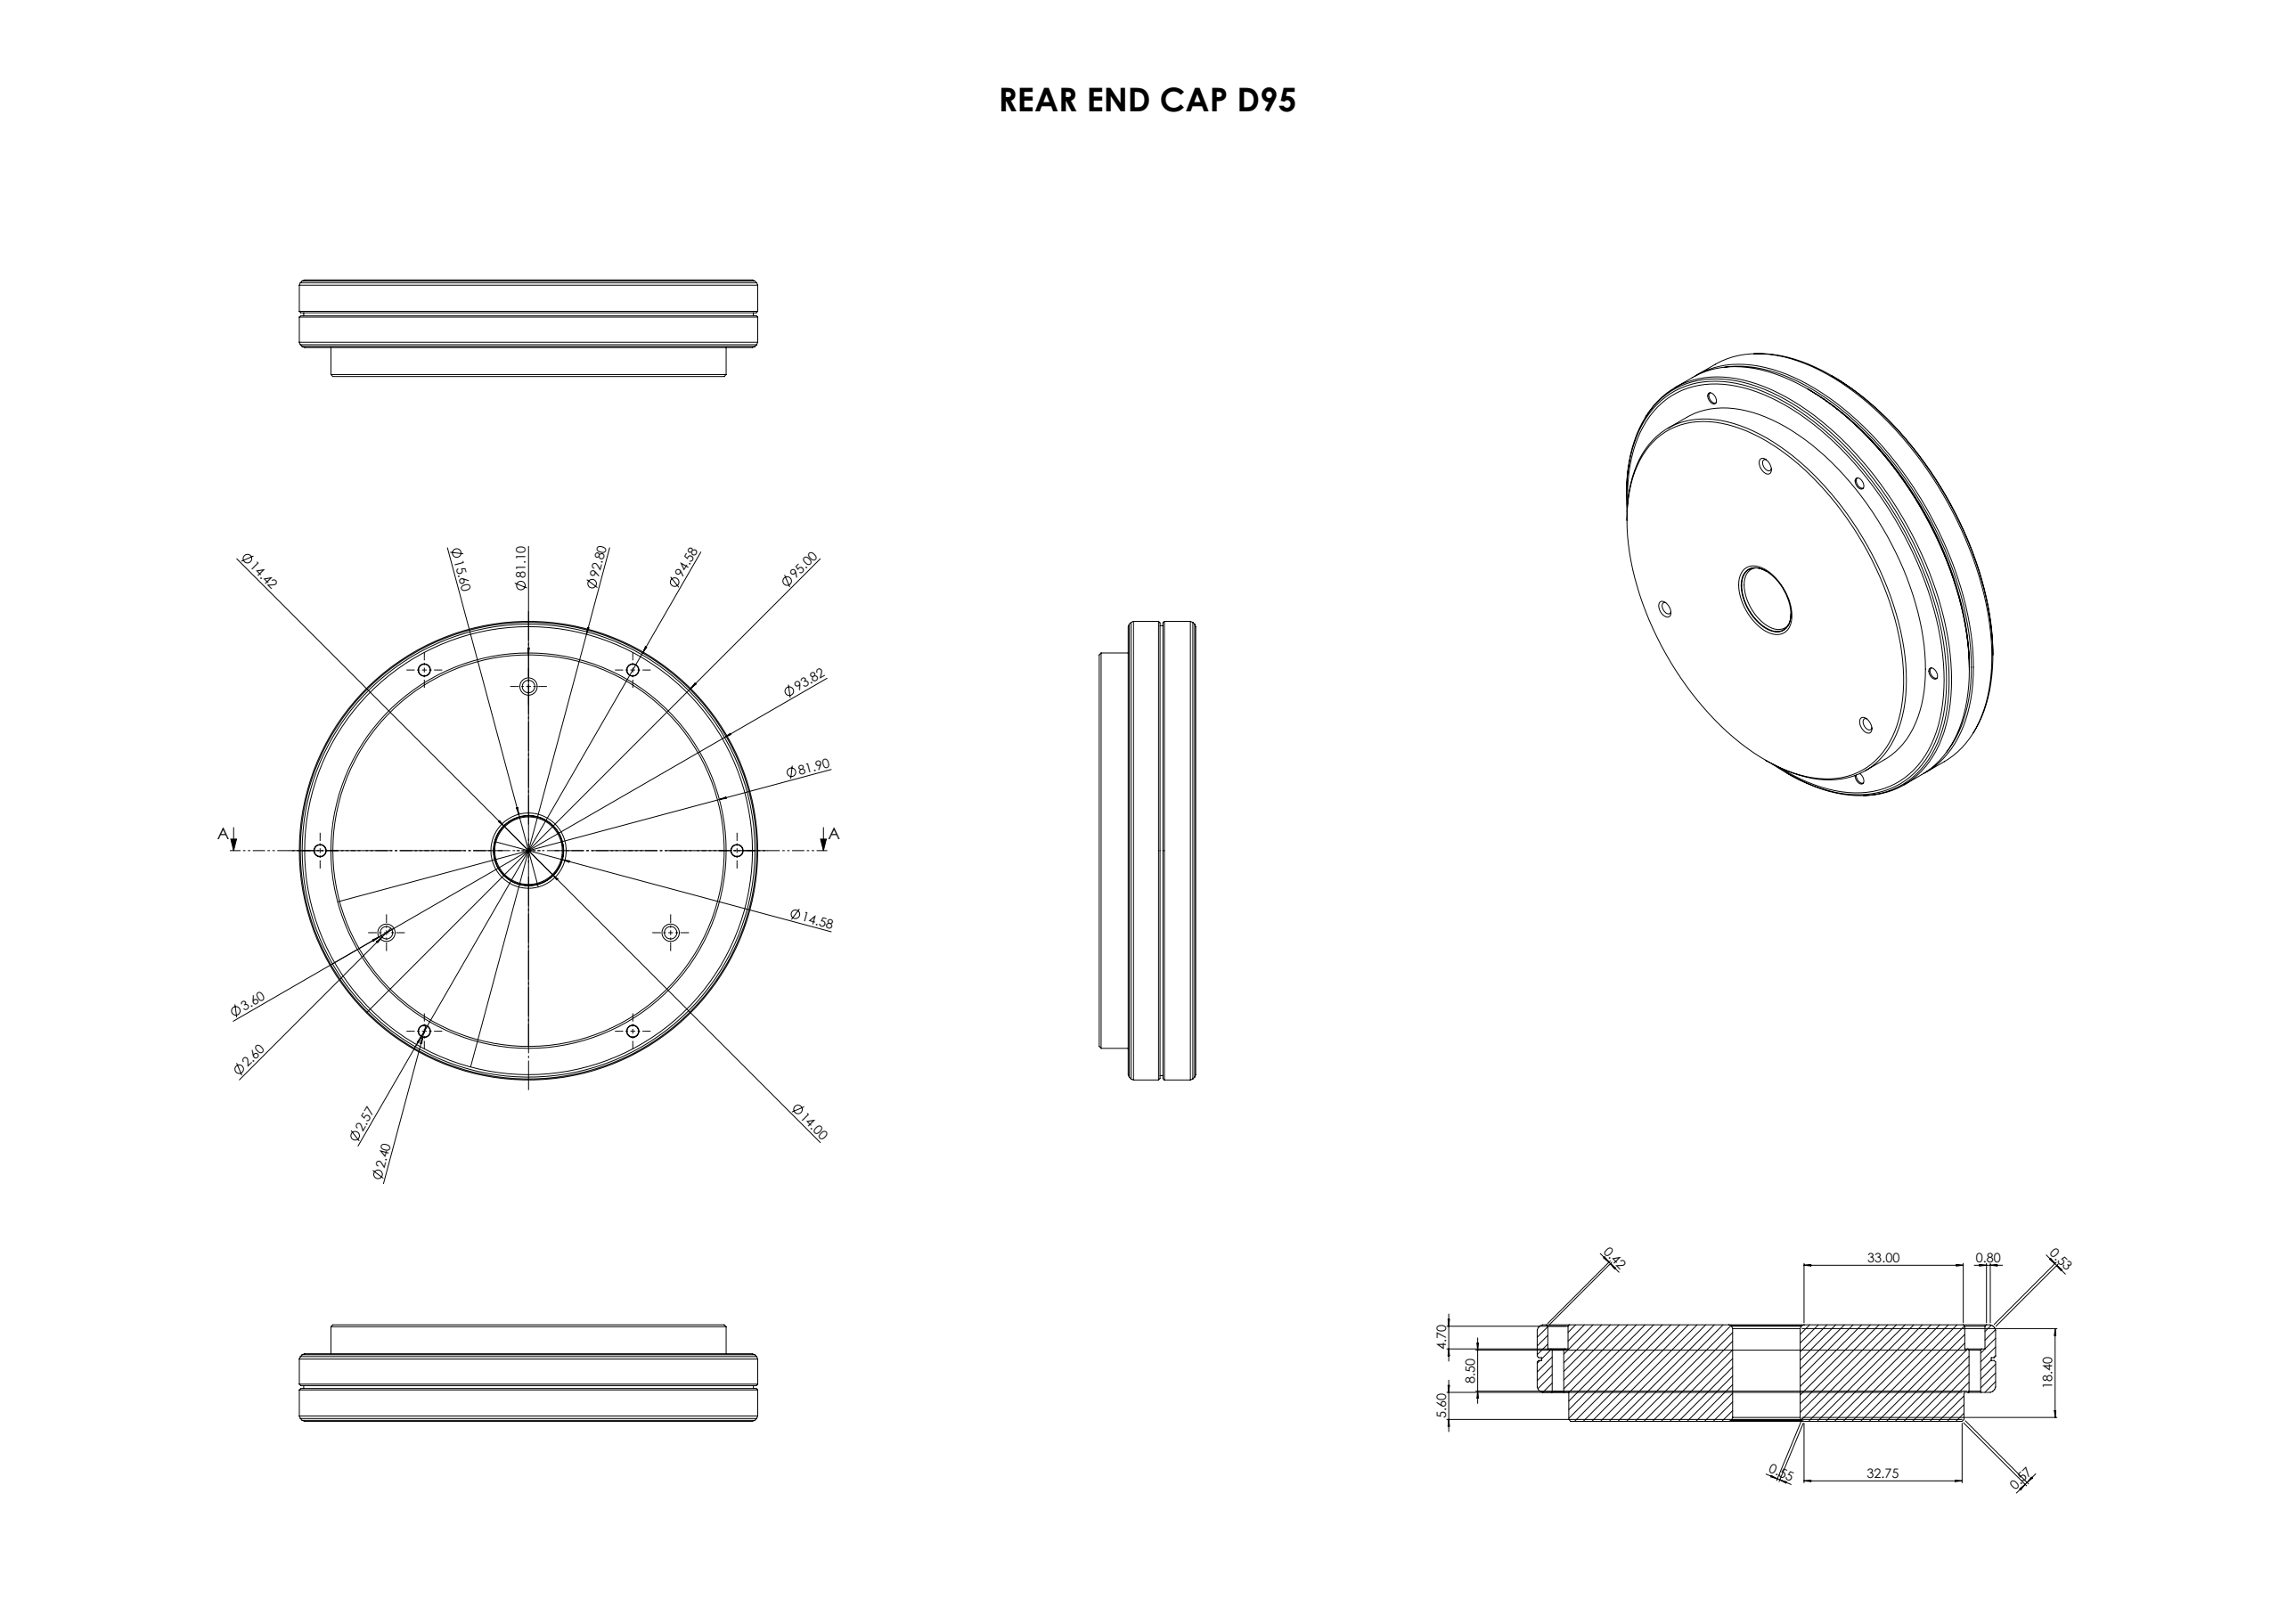
ISO-10303-21;
HEADER;
/* Generated by software containing ST-Developer
 * from STEP Tools, Inc. (www.steptools.com) 
 */

FILE_DESCRIPTION(
/* description */ (''),
/* implementation_level */ '2;1');

FILE_NAME(
/* name */ '01_Rear_End_Cap_D95.step',
/* time_stamp */ '2026-10-19T23:00:43-07:00',
/* author */ (''),
/* organization */ (''),
/* preprocessor_version */ 'ST-DEVELOPER v20.2',
/* originating_system */ 'Autodesk Translation Framework v15.15.0.0',
/* authorisation */ '');

FILE_SCHEMA (('AUTOMOTIVE_DESIGN { 1 0 10303 214 3 1 1 }'));
ENDSEC;

DATA;
#10=MECHANICAL_DESIGN_GEOMETRIC_PRESENTATION_REPRESENTATION('',(#996),#55002);
#956=SHAPE_REPRESENTATION_RELATIONSHIP('SRR','None',#55104,#976);
#976=ADVANCED_BREP_SHAPE_REPRESENTATION('',(#1016),#54982);
#996=STYLED_ITEM('',(#55372),#1016);
#1016=MANIFOLD_SOLID_BREP('Rear End Cap',#24529);
#1036=FACE_BOUND('',#3782,.T.);
#1037=FACE_BOUND('',#3783,.T.);
#1038=FACE_BOUND('',#3784,.T.);
#1039=FACE_BOUND('',#3785,.T.);
#1040=FACE_BOUND('',#3786,.T.);
#1041=FACE_BOUND('',#3787,.T.);
#1042=FACE_BOUND('',#3788,.T.);
#1043=FACE_BOUND('',#3791,.T.);
#1044=FACE_BOUND('',#3792,.T.);
#1045=FACE_BOUND('',#3793,.T.);
#1046=FACE_BOUND('',#3794,.T.);
#1047=FACE_BOUND('',#3795,.T.);
#1048=FACE_BOUND('',#3796,.T.);
#1049=FACE_BOUND('',#3797,.T.);
#1050=FACE_BOUND('',#3806,.T.);
#1051=FACE_BOUND('',#3807,.T.);
#1052=FACE_BOUND('',#3808,.T.);
#1053=FACE_BOUND('',#3809,.T.);
#1054=FACE_BOUND('',#3826,.T.);
#1055=FACE_BOUND('',#3829,.T.);
#1056=FACE_BOUND('',#3844,.T.);
#1057=FACE_BOUND('',#3849,.T.);
#1058=FACE_BOUND('',#3854,.T.);
#1059=FACE_BOUND('',#3859,.T.);
#1060=FACE_BOUND('',#3864,.T.);
#1061=FACE_BOUND('',#3869,.T.);
#1276=PLANE('',#24785);
#1277=PLANE('',#24795);
#1278=PLANE('',#24819);
#1279=PLANE('',#24861);
#1280=PLANE('',#24865);
#1281=PLANE('',#24889);
#1282=PLANE('',#24896);
#1283=PLANE('',#24903);
#1284=PLANE('',#24910);
#1285=PLANE('',#24917);
#1286=PLANE('',#24924);
#1952=CYLINDRICAL_SURFACE('',#24778,4.75);
#1953=CYLINDRICAL_SURFACE('',#24810,0.7);
#1954=CYLINDRICAL_SURFACE('',#24827,0.21);
#1955=CYLINDRICAL_SURFACE('',#24832,0.21);
#1956=CYLINDRICAL_SURFACE('',#24837,0.21);
#1957=CYLINDRICAL_SURFACE('',#24842,0.21);
#1958=CYLINDRICAL_SURFACE('',#24847,0.21);
#1959=CYLINDRICAL_SURFACE('',#24852,0.21);
#1960=CYLINDRICAL_SURFACE('',#24857,4.75);
#1961=CYLINDRICAL_SURFACE('',#24867,4.66);
#1962=CYLINDRICAL_SURFACE('',#24870,0.13);
#1963=CYLINDRICAL_SURFACE('',#24875,0.13);
#1964=CYLINDRICAL_SURFACE('',#24880,0.13);
#1965=CYLINDRICAL_SURFACE('',#24885,0.12);
#1966=CYLINDRICAL_SURFACE('',#24892,0.12);
#1967=CYLINDRICAL_SURFACE('',#24899,0.12);
#1968=CYLINDRICAL_SURFACE('',#24906,0.12);
#1969=CYLINDRICAL_SURFACE('',#24913,0.12);
#1970=CYLINDRICAL_SURFACE('',#24920,0.12);
#1971=CYLINDRICAL_SURFACE('',#24928,4.095);
#2412=FACE_OUTER_BOUND('',#3776,.T.);
#2413=FACE_OUTER_BOUND('',#3777,.T.);
#2414=FACE_OUTER_BOUND('',#3778,.T.);
#2415=FACE_OUTER_BOUND('',#3779,.T.);
#2416=FACE_OUTER_BOUND('',#3780,.T.);
#2417=FACE_OUTER_BOUND('',#3781,.T.);
#2418=FACE_OUTER_BOUND('',#3789,.T.);
#2419=FACE_OUTER_BOUND('',#3790,.T.);
#2420=FACE_OUTER_BOUND('',#3798,.T.);
#2421=FACE_OUTER_BOUND('',#3799,.T.);
#2422=FACE_OUTER_BOUND('',#3800,.T.);
#2423=FACE_OUTER_BOUND('',#3801,.T.);
#2424=FACE_OUTER_BOUND('',#3802,.T.);
#2425=FACE_OUTER_BOUND('',#3803,.T.);
#2426=FACE_OUTER_BOUND('',#3804,.T.);
#2427=FACE_OUTER_BOUND('',#3805,.T.);
#2428=FACE_OUTER_BOUND('',#3810,.T.);
#2429=FACE_OUTER_BOUND('',#3811,.T.);
#2430=FACE_OUTER_BOUND('',#3812,.T.);
#2431=FACE_OUTER_BOUND('',#3813,.T.);
#2432=FACE_OUTER_BOUND('',#3814,.T.);
#2433=FACE_OUTER_BOUND('',#3815,.T.);
#2434=FACE_OUTER_BOUND('',#3816,.T.);
#2435=FACE_OUTER_BOUND('',#3817,.T.);
#2436=FACE_OUTER_BOUND('',#3818,.T.);
#2437=FACE_OUTER_BOUND('',#3819,.T.);
#2438=FACE_OUTER_BOUND('',#3820,.T.);
#2439=FACE_OUTER_BOUND('',#3821,.T.);
#2440=FACE_OUTER_BOUND('',#3822,.T.);
#2441=FACE_OUTER_BOUND('',#3823,.T.);
#2442=FACE_OUTER_BOUND('',#3824,.T.);
#2443=FACE_OUTER_BOUND('',#3825,.T.);
#2444=FACE_OUTER_BOUND('',#3827,.T.);
#2445=FACE_OUTER_BOUND('',#3828,.T.);
#2446=FACE_OUTER_BOUND('',#3830,.T.);
#2447=FACE_OUTER_BOUND('',#3831,.T.);
#2448=FACE_OUTER_BOUND('',#3832,.T.);
#2449=FACE_OUTER_BOUND('',#3833,.T.);
#2450=FACE_OUTER_BOUND('',#3834,.T.);
#2451=FACE_OUTER_BOUND('',#3835,.T.);
#2452=FACE_OUTER_BOUND('',#3836,.T.);
#2453=FACE_OUTER_BOUND('',#3837,.T.);
#2454=FACE_OUTER_BOUND('',#3838,.T.);
#2455=FACE_OUTER_BOUND('',#3839,.T.);
#2456=FACE_OUTER_BOUND('',#3840,.T.);
#2457=FACE_OUTER_BOUND('',#3841,.T.);
#2458=FACE_OUTER_BOUND('',#3842,.T.);
#2459=FACE_OUTER_BOUND('',#3843,.T.);
#2460=FACE_OUTER_BOUND('',#3845,.T.);
#2461=FACE_OUTER_BOUND('',#3846,.T.);
#2462=FACE_OUTER_BOUND('',#3847,.T.);
#2463=FACE_OUTER_BOUND('',#3848,.T.);
#2464=FACE_OUTER_BOUND('',#3850,.T.);
#2465=FACE_OUTER_BOUND('',#3851,.T.);
#2466=FACE_OUTER_BOUND('',#3852,.T.);
#2467=FACE_OUTER_BOUND('',#3853,.T.);
#2468=FACE_OUTER_BOUND('',#3855,.T.);
#2469=FACE_OUTER_BOUND('',#3856,.T.);
#2470=FACE_OUTER_BOUND('',#3857,.T.);
#2471=FACE_OUTER_BOUND('',#3858,.T.);
#2472=FACE_OUTER_BOUND('',#3860,.T.);
#2473=FACE_OUTER_BOUND('',#3861,.T.);
#2474=FACE_OUTER_BOUND('',#3862,.T.);
#2475=FACE_OUTER_BOUND('',#3863,.T.);
#2476=FACE_OUTER_BOUND('',#3865,.T.);
#2477=FACE_OUTER_BOUND('',#3866,.T.);
#2478=FACE_OUTER_BOUND('',#3867,.T.);
#2479=FACE_OUTER_BOUND('',#3868,.T.);
#2480=FACE_OUTER_BOUND('',#3870,.T.);
#2481=FACE_OUTER_BOUND('',#3871,.T.);
#3776=EDGE_LOOP('',(#15886,#15887,#15888,#15889,#15890));
#3777=EDGE_LOOP('',(#15891,#15892,#15893,#15894));
#3778=EDGE_LOOP('',(#15895,#15896,#15897,#15898,#15899));
#3779=EDGE_LOOP('',(#15900,#15901,#15902,#15903));
#3780=EDGE_LOOP('',(#15904,#15905,#15906,#15907));
#3781=EDGE_LOOP('',(#15908));
#3782=EDGE_LOOP('',(#15909));
#3783=EDGE_LOOP('',(#15910));
#3784=EDGE_LOOP('',(#15911));
#3785=EDGE_LOOP('',(#15912));
#3786=EDGE_LOOP('',(#15913));
#3787=EDGE_LOOP('',(#15914));
#3788=EDGE_LOOP('',(#15915));
#3789=EDGE_LOOP('',(#15916,#15917,#15918,#15919));
#3790=EDGE_LOOP('',(#15920));
#3791=EDGE_LOOP('',(#15921));
#3792=EDGE_LOOP('',(#15922));
#3793=EDGE_LOOP('',(#15923));
#3794=EDGE_LOOP('',(#15924));
#3795=EDGE_LOOP('',(#15925));
#3796=EDGE_LOOP('',(#15926));
#3797=EDGE_LOOP('',(#15927));
#3798=EDGE_LOOP('',(#15928,#15929,#15930,#15931));
#3799=EDGE_LOOP('',(#15932,#15933,#15934,#15935));
#3800=EDGE_LOOP('',(#15936,#15937,#15938,#15939,#15940));
#3801=EDGE_LOOP('',(#15941,#15942,#15943,#15944,#15945,#15946));
#3802=EDGE_LOOP('',(#15947,#15948,#15949,#15950,#15951));
#3803=EDGE_LOOP('',(#15952,#15953,#15954,#15955));
#3804=EDGE_LOOP('',(#15956,#15957,#15958,#15959));
#3805=EDGE_LOOP('',(#15960));
#3806=EDGE_LOOP('',(#15961));
#3807=EDGE_LOOP('',(#15962));
#3808=EDGE_LOOP('',(#15963));
#3809=EDGE_LOOP('',(#15964));
#3810=EDGE_LOOP('',(#15965,#15966,#15967,#15968,#15969));
#3811=EDGE_LOOP('',(#15970,#15971,#15972,#15973,#15974));
#3812=EDGE_LOOP('',(#15975,#15976,#15977,#15978,#15979));
#3813=EDGE_LOOP('',(#15980,#15981,#15982,#15983,#15984));
#3814=EDGE_LOOP('',(#15985,#15986,#15987,#15988,#15989));
#3815=EDGE_LOOP('',(#15990,#15991,#15992,#15993,#15994));
#3816=EDGE_LOOP('',(#15995,#15996,#15997,#15998,#15999));
#3817=EDGE_LOOP('',(#16000,#16001,#16002,#16003,#16004));
#3818=EDGE_LOOP('',(#16005,#16006,#16007,#16008,#16009));
#3819=EDGE_LOOP('',(#16010,#16011,#16012,#16013,#16014));
#3820=EDGE_LOOP('',(#16015,#16016,#16017,#16018,#16019));
#3821=EDGE_LOOP('',(#16020,#16021,#16022,#16023,#16024));
#3822=EDGE_LOOP('',(#16025,#16026,#16027,#16028,#16029));
#3823=EDGE_LOOP('',(#16030,#16031,#16032,#16033,#16034));
#3824=EDGE_LOOP('',(#16035,#16036,#16037,#16038));
#3825=EDGE_LOOP('',(#16039));
#3826=EDGE_LOOP('',(#16040));
#3827=EDGE_LOOP('',(#16041,#16042,#16043,#16044));
#3828=EDGE_LOOP('',(#16045));
#3829=EDGE_LOOP('',(#16046));
#3830=EDGE_LOOP('',(#16047,#16048,#16049,#16050));
#3831=EDGE_LOOP('',(#16051,#16052,#16053));
#3832=EDGE_LOOP('',(#16054,#16055,#16056,#16057));
#3833=EDGE_LOOP('',(#16058,#16059,#16060,#16061));
#3834=EDGE_LOOP('',(#16062,#16063,#16064));
#3835=EDGE_LOOP('',(#16065,#16066,#16067,#16068));
#3836=EDGE_LOOP('',(#16069,#16070,#16071,#16072));
#3837=EDGE_LOOP('',(#16073,#16074,#16075));
#3838=EDGE_LOOP('',(#16076,#16077,#16078,#16079));
#3839=EDGE_LOOP('',(#16080,#16081,#16082,#16083));
#3840=EDGE_LOOP('',(#16084,#16085,#16086,#16087));
#3841=EDGE_LOOP('',(#16088,#16089,#16090,#16091));
#3842=EDGE_LOOP('',(#16092,#16093,#16094,#16095));
#3843=EDGE_LOOP('',(#16096));
#3844=EDGE_LOOP('',(#16097));
#3845=EDGE_LOOP('',(#16098,#16099,#16100,#16101));
#3846=EDGE_LOOP('',(#16102,#16103,#16104,#16105));
#3847=EDGE_LOOP('',(#16106,#16107,#16108,#16109));
#3848=EDGE_LOOP('',(#16110));
#3849=EDGE_LOOP('',(#16111));
#3850=EDGE_LOOP('',(#16112,#16113,#16114,#16115));
#3851=EDGE_LOOP('',(#16116,#16117,#16118,#16119));
#3852=EDGE_LOOP('',(#16120,#16121,#16122,#16123));
#3853=EDGE_LOOP('',(#16124));
#3854=EDGE_LOOP('',(#16125));
#3855=EDGE_LOOP('',(#16126,#16127,#16128,#16129));
#3856=EDGE_LOOP('',(#16130,#16131,#16132,#16133));
#3857=EDGE_LOOP('',(#16134,#16135,#16136,#16137));
#3858=EDGE_LOOP('',(#16138));
#3859=EDGE_LOOP('',(#16139));
#3860=EDGE_LOOP('',(#16140,#16141,#16142,#16143));
#3861=EDGE_LOOP('',(#16144,#16145,#16146,#16147));
#3862=EDGE_LOOP('',(#16148,#16149,#16150,#16151));
#3863=EDGE_LOOP('',(#16152));
#3864=EDGE_LOOP('',(#16153));
#3865=EDGE_LOOP('',(#16154,#16155,#16156,#16157));
#3866=EDGE_LOOP('',(#16158,#16159,#16160,#16161));
#3867=EDGE_LOOP('',(#16162,#16163,#16164,#16165));
#3868=EDGE_LOOP('',(#16166));
#3869=EDGE_LOOP('',(#16167));
#3870=EDGE_LOOP('',(#16168,#16169,#16170,#16171,#16172));
#3871=EDGE_LOOP('',(#16173,#16174,#16175,#16176,#16177));
#5380=LINE('',#33875,#7201);
#5381=LINE('',#33881,#7202);
#5382=LINE('',#33886,#7203);
#5383=LINE('',#33891,#7204);
#5384=LINE('',#33895,#7205);
#5385=LINE('',#33914,#7206);
#5386=LINE('',#33934,#7207);
#5387=LINE('',#33937,#7208);
#5388=LINE('',#33941,#7209);
#5389=LINE('',#33950,#7210);
#5390=LINE('',#33954,#7211);
#5391=LINE('',#33957,#7212);
#5392=LINE('',#33961,#7213);
#5393=LINE('',#33974,#7214);
#5394=LINE('',#33981,#7215);
#5395=LINE('',#33984,#7216);
#5396=LINE('',#33991,#7217);
#5397=LINE('',#33994,#7218);
#5398=LINE('',#34001,#7219);
#5399=LINE('',#34004,#7220);
#5400=LINE('',#34011,#7221);
#5401=LINE('',#34014,#7222);
#5402=LINE('',#34021,#7223);
#5403=LINE('',#34024,#7224);
#5404=LINE('',#34031,#7225);
#5405=LINE('',#34034,#7226);
#5406=LINE('',#34040,#7227);
#5407=LINE('',#34044,#7228);
#5408=LINE('',#34051,#7229);
#5409=LINE('',#34057,#7230);
#5410=LINE('',#34061,#7231);
#5411=LINE('',#34065,#7232);
#5412=LINE('',#34068,#7233);
#5413=LINE('',#34072,#7234);
#5414=LINE('',#34076,#7235);
#5415=LINE('',#34079,#7236);
#5416=LINE('',#34083,#7237);
#5417=LINE('',#34087,#7238);
#5418=LINE('',#34090,#7239);
#5419=LINE('',#34093,#7240);
#5420=LINE('',#34097,#7241);
#5421=LINE('',#34101,#7242);
#5422=LINE('',#34106,#7243);
#5423=LINE('',#34110,#7244);
#5424=LINE('',#34114,#7245);
#5425=LINE('',#34119,#7246);
#5426=LINE('',#34123,#7247);
#5427=LINE('',#34127,#7248);
#5428=LINE('',#34132,#7249);
#5429=LINE('',#34136,#7250);
#5430=LINE('',#34140,#7251);
#5431=LINE('',#34145,#7252);
#5432=LINE('',#34149,#7253);
#5433=LINE('',#34153,#7254);
#5434=LINE('',#34158,#7255);
#5435=LINE('',#34162,#7256);
#5436=LINE('',#34166,#7257);
#5437=LINE('',#34171,#7258);
#5438=LINE('',#34176,#7259);
#7201=VECTOR('',#27204,4.7393933982822);
#7202=VECTOR('',#27211,4.71);
#7203=VECTOR('',#27218,4.75);
#7204=VECTOR('',#27223,4.6656066017178);
#7205=VECTOR('',#27228,4.71);
#7206=VECTOR('',#27249,4.6656066017178);
#7207=VECTOR('',#27272,0.754393398282202);
#7208=VECTOR('',#27275,0.725);
#7209=VECTOR('',#27280,0.710606601717798);
#7210=VECTOR('',#27291,0.7);
#7211=VECTOR('',#27296,0.710606601717798);
#7212=VECTOR('',#27299,0.725);
#7213=VECTOR('',#27304,0.754393398282202);
#7214=VECTOR('',#27319,0.225);
#7215=VECTOR('',#27328,0.21);
#7216=VECTOR('',#27331,0.225);
#7217=VECTOR('',#27340,0.21);
#7218=VECTOR('',#27343,0.225);
#7219=VECTOR('',#27352,0.21);
#7220=VECTOR('',#27355,0.225);
#7221=VECTOR('',#27364,0.21);
#7222=VECTOR('',#27367,0.225);
#7223=VECTOR('',#27376,0.21);
#7224=VECTOR('',#27379,0.225);
#7225=VECTOR('',#27388,0.21);
#7226=VECTOR('',#27391,4.7393933982822);
#7227=VECTOR('',#27398,4.75);
#7228=VECTOR('',#27403,4.735);
#7229=VECTOR('',#27412,4.735);
#7230=VECTOR('',#27421,4.66);
#7231=VECTOR('',#27424,0.0649999999999999);
#7232=VECTOR('',#27429,0.13);
#7233=VECTOR('',#27434,0.18);
#7234=VECTOR('',#27437,0.0649999999999999);
#7235=VECTOR('',#27442,0.13);
#7236=VECTOR('',#27447,0.18);
#7237=VECTOR('',#27450,0.065);
#7238=VECTOR('',#27455,0.13);
#7239=VECTOR('',#27460,0.18);
#7240=VECTOR('',#27463,0.1325);
#7241=VECTOR('',#27468,0.12);
#7242=VECTOR('',#27473,0.1325);
#7243=VECTOR('',#27480,0.1325);
#7244=VECTOR('',#27485,0.12);
#7245=VECTOR('',#27490,0.1325);
#7246=VECTOR('',#27497,0.1325);
#7247=VECTOR('',#27502,0.12);
#7248=VECTOR('',#27507,0.1325);
#7249=VECTOR('',#27514,0.132499999999999);
#7250=VECTOR('',#27519,0.12);
#7251=VECTOR('',#27524,0.132499999999999);
#7252=VECTOR('',#27531,0.1325);
#7253=VECTOR('',#27536,0.12);
#7254=VECTOR('',#27541,0.1325);
#7255=VECTOR('',#27548,0.1325);
#7256=VECTOR('',#27553,0.12);
#7257=VECTOR('',#27558,0.1325);
#7258=VECTOR('',#27565,4.075);
#7259=VECTOR('',#27572,4.095);
#9022=CIRCLE('',#24773,4.7287867965644);
#9023=CIRCLE('',#24774,4.75);
#9024=CIRCLE('',#24775,4.75);
#9025=CIRCLE('',#24777,4.6912132034356);
#9026=CIRCLE('',#24779,4.75);
#9027=CIRCLE('',#24781,4.6912132034356);
#9028=CIRCLE('',#24782,4.64);
#9029=CIRCLE('',#24784,4.7287867965644);
#9030=CIRCLE('',#24786,4.095);
#9031=CIRCLE('',#24787,0.128333333333333);
#9032=CIRCLE('',#24788,0.128333333333333);
#9033=CIRCLE('',#24789,0.128333333333333);
#9034=CIRCLE('',#24790,0.128333333333333);
#9035=CIRCLE('',#24791,0.128333333333334);
#9036=CIRCLE('',#24792,0.128333333333333);
#9037=CIRCLE('',#24794,4.64);
#9038=CIRCLE('',#24796,0.78);
#9039=CIRCLE('',#24797,0.24);
#9040=CIRCLE('',#24798,0.24);
#9041=CIRCLE('',#24799,0.24);
#9042=CIRCLE('',#24800,0.24);
#9043=CIRCLE('',#24801,0.24);
#9044=CIRCLE('',#24802,0.24);
#9045=CIRCLE('',#24804,0.728786796564404);
#9046=CIRCLE('',#24806,0.721213203435596);
#9047=CIRCLE('',#24808,0.7);
#9048=CIRCLE('',#24809,0.7);
#9049=CIRCLE('',#24811,0.7);
#9050=CIRCLE('',#24812,0.7);
#9051=CIRCLE('',#24814,0.721213203435596);
#9052=CIRCLE('',#24816,0.728786796564404);
#9053=CIRCLE('',#24818,0.78);
#9054=CIRCLE('',#24820,4.055);
#9055=CIRCLE('',#24821,0.18);
#9056=CIRCLE('',#24822,0.18);
#9057=CIRCLE('',#24823,0.18);
#9058=CIRCLE('',#24825,0.21);
#9059=CIRCLE('',#24826,0.21);
#9060=CIRCLE('',#24828,0.21);
#9061=CIRCLE('',#24830,0.21);
#9062=CIRCLE('',#24831,0.21);
#9063=CIRCLE('',#24833,0.21);
#9064=CIRCLE('',#24835,0.21);
#9065=CIRCLE('',#24836,0.21);
#9066=CIRCLE('',#24838,0.21);
#9067=CIRCLE('',#24840,0.21);
#9068=CIRCLE('',#24841,0.21);
#9069=CIRCLE('',#24843,0.21);
#9070=CIRCLE('',#24845,0.21);
#9071=CIRCLE('',#24846,0.21);
#9072=CIRCLE('',#24848,0.21);
#9073=CIRCLE('',#24850,0.21);
#9074=CIRCLE('',#24851,0.21);
#9075=CIRCLE('',#24853,0.21);
#9076=CIRCLE('',#24855,4.75);
#9077=CIRCLE('',#24856,4.75);
#9078=CIRCLE('',#24858,4.75);
#9079=CIRCLE('',#24860,4.72);
#9080=CIRCLE('',#24862,4.66);
#9081=CIRCLE('',#24864,4.72);
#9082=CIRCLE('',#24866,4.66);
#9083=CIRCLE('',#24869,0.13);
#9084=CIRCLE('',#24871,0.13);
#9085=CIRCLE('',#24874,0.13);
#9086=CIRCLE('',#24876,0.13);
#9087=CIRCLE('',#24879,0.13);
#9088=CIRCLE('',#24881,0.13);
#9089=CIRCLE('',#24884,0.12);
#9090=CIRCLE('',#24886,0.12);
#9091=CIRCLE('',#24888,0.145);
#9092=CIRCLE('',#24891,0.12);
#9093=CIRCLE('',#24893,0.12);
#9094=CIRCLE('',#24895,0.145);
#9095=CIRCLE('',#24898,0.12);
#9096=CIRCLE('',#24900,0.12);
#9097=CIRCLE('',#24902,0.145);
#9098=CIRCLE('',#24905,0.12);
#9099=CIRCLE('',#24907,0.12);
#9100=CIRCLE('',#24909,0.145);
#9101=CIRCLE('',#24912,0.12);
#9102=CIRCLE('',#24914,0.12);
#9103=CIRCLE('',#24916,0.145);
#9104=CIRCLE('',#24919,0.12);
#9105=CIRCLE('',#24921,0.12);
#9106=CIRCLE('',#24923,0.145);
#9107=CIRCLE('',#24926,4.095);
#9108=CIRCLE('',#24927,4.095);
#10026=VERTEX_POINT('',#33872);
#10027=VERTEX_POINT('',#33874);
#10028=VERTEX_POINT('',#33876);
#10029=VERTEX_POINT('',#33880);
#10030=VERTEX_POINT('',#33884);
#10031=VERTEX_POINT('',#33888);
#10032=VERTEX_POINT('',#33890);
#10033=VERTEX_POINT('',#33894);
#10034=VERTEX_POINT('',#33898);
#10035=VERTEX_POINT('',#33900);
#10036=VERTEX_POINT('',#33902);
#10037=VERTEX_POINT('',#33904);
#10038=VERTEX_POINT('',#33906);
#10039=VERTEX_POINT('',#33908);
#10040=VERTEX_POINT('',#33910);
#10041=VERTEX_POINT('',#33913);
#10042=VERTEX_POINT('',#33917);
#10043=VERTEX_POINT('',#33919);
#10044=VERTEX_POINT('',#33921);
#10045=VERTEX_POINT('',#33923);
#10046=VERTEX_POINT('',#33925);
#10047=VERTEX_POINT('',#33927);
#10048=VERTEX_POINT('',#33929);
#10049=VERTEX_POINT('',#33932);
#10050=VERTEX_POINT('',#33936);
#10051=VERTEX_POINT('',#33940);
#10052=VERTEX_POINT('',#33942);
#10053=VERTEX_POINT('',#33946);
#10054=VERTEX_POINT('',#33947);
#10055=VERTEX_POINT('',#33952);
#10056=VERTEX_POINT('',#33956);
#10057=VERTEX_POINT('',#33960);
#10058=VERTEX_POINT('',#33964);
#10059=VERTEX_POINT('',#33966);
#10060=VERTEX_POINT('',#33968);
#10061=VERTEX_POINT('',#33970);
#10062=VERTEX_POINT('',#33973);
#10063=VERTEX_POINT('',#33975);
#10064=VERTEX_POINT('',#33979);
#10065=VERTEX_POINT('',#33983);
#10066=VERTEX_POINT('',#33985);
#10067=VERTEX_POINT('',#33989);
#10068=VERTEX_POINT('',#33993);
#10069=VERTEX_POINT('',#33995);
#10070=VERTEX_POINT('',#33999);
#10071=VERTEX_POINT('',#34003);
#10072=VERTEX_POINT('',#34005);
#10073=VERTEX_POINT('',#34009);
#10074=VERTEX_POINT('',#34013);
#10075=VERTEX_POINT('',#34015);
#10076=VERTEX_POINT('',#34019);
#10077=VERTEX_POINT('',#34023);
#10078=VERTEX_POINT('',#34025);
#10079=VERTEX_POINT('',#34029);
#10080=VERTEX_POINT('',#34033);
#10081=VERTEX_POINT('',#34035);
#10082=VERTEX_POINT('',#34039);
#10083=VERTEX_POINT('',#34043);
#10084=VERTEX_POINT('',#34047);
#10085=VERTEX_POINT('',#34050);
#10086=VERTEX_POINT('',#34054);
#10087=VERTEX_POINT('',#34059);
#10088=VERTEX_POINT('',#34060);
#10089=VERTEX_POINT('',#34064);
#10090=VERTEX_POINT('',#34070);
#10091=VERTEX_POINT('',#34071);
#10092=VERTEX_POINT('',#34075);
#10093=VERTEX_POINT('',#34081);
#10094=VERTEX_POINT('',#34082);
#10095=VERTEX_POINT('',#34086);
#10096=VERTEX_POINT('',#34092);
#10097=VERTEX_POINT('',#34096);
#10098=VERTEX_POINT('',#34100);
#10099=VERTEX_POINT('',#34105);
#10100=VERTEX_POINT('',#34109);
#10101=VERTEX_POINT('',#34113);
#10102=VERTEX_POINT('',#34118);
#10103=VERTEX_POINT('',#34122);
#10104=VERTEX_POINT('',#34126);
#10105=VERTEX_POINT('',#34131);
#10106=VERTEX_POINT('',#34135);
#10107=VERTEX_POINT('',#34139);
#10108=VERTEX_POINT('',#34144);
#10109=VERTEX_POINT('',#34148);
#10110=VERTEX_POINT('',#34152);
#10111=VERTEX_POINT('',#34157);
#10112=VERTEX_POINT('',#34161);
#10113=VERTEX_POINT('',#34165);
#10114=VERTEX_POINT('',#34170);
#10115=VERTEX_POINT('',#34172);
#12351=EDGE_CURVE('',#10026,#10026,#9022,.T.);
#12352=EDGE_CURVE('',#10026,#10027,#5380,.T.);
#12353=EDGE_CURVE('',#10027,#10028,#9023,.T.);
#12354=EDGE_CURVE('',#10028,#10027,#9024,.T.);
#12355=EDGE_CURVE('',#10026,#10029,#5381,.T.);
#12356=EDGE_CURVE('',#10029,#10029,#9025,.T.);
#12357=EDGE_CURVE('',#10030,#10030,#9026,.T.);
#12358=EDGE_CURVE('',#10030,#10028,#5382,.T.);
#12359=EDGE_CURVE('',#10031,#10031,#9027,.T.);
#12360=EDGE_CURVE('',#10031,#10032,#5383,.T.);
#12361=EDGE_CURVE('',#10032,#10032,#9028,.T.);
#12362=EDGE_CURVE('',#10031,#10033,#5384,.T.);
#12363=EDGE_CURVE('',#10033,#10033,#9029,.T.);
#12364=EDGE_CURVE('',#10034,#10034,#9030,.T.);
#12365=EDGE_CURVE('',#10035,#10035,#9031,.T.);
#12366=EDGE_CURVE('',#10036,#10036,#9032,.T.);
#12367=EDGE_CURVE('',#10037,#10037,#9033,.T.);
#12368=EDGE_CURVE('',#10038,#10038,#9034,.T.);
#12369=EDGE_CURVE('',#10039,#10039,#9035,.T.);
#12370=EDGE_CURVE('',#10040,#10040,#9036,.T.);
#12371=EDGE_CURVE('',#10029,#10041,#5385,.T.);
#12372=EDGE_CURVE('',#10041,#10041,#9037,.T.);
#12373=EDGE_CURVE('',#10042,#10042,#9038,.T.);
#12374=EDGE_CURVE('',#10043,#10043,#9039,.T.);
#12375=EDGE_CURVE('',#10044,#10044,#9040,.T.);
#12376=EDGE_CURVE('',#10045,#10045,#9041,.T.);
#12377=EDGE_CURVE('',#10046,#10046,#9042,.T.);
#12378=EDGE_CURVE('',#10047,#10047,#9043,.T.);
#12379=EDGE_CURVE('',#10048,#10048,#9044,.T.);
#12380=EDGE_CURVE('',#10049,#10049,#9045,.T.);
#12381=EDGE_CURVE('',#10049,#10042,#5386,.T.);
#12382=EDGE_CURVE('',#10049,#10050,#5387,.T.);
#12383=EDGE_CURVE('',#10050,#10050,#9046,.T.);
#12384=EDGE_CURVE('',#10050,#10051,#5388,.T.);
#12385=EDGE_CURVE('',#10051,#10052,#9047,.T.);
#12386=EDGE_CURVE('',#10052,#10051,#9048,.T.);
#12387=EDGE_CURVE('',#10053,#10054,#9049,.T.);
#12388=EDGE_CURVE('',#10054,#10053,#9050,.T.);
#12389=EDGE_CURVE('',#10054,#10052,#5389,.T.);
#12390=EDGE_CURVE('',#10055,#10055,#9051,.T.);
#12391=EDGE_CURVE('',#10055,#10053,#5390,.T.);
#12392=EDGE_CURVE('',#10055,#10056,#5391,.T.);
#12393=EDGE_CURVE('',#10056,#10056,#9052,.T.);
#12394=EDGE_CURVE('',#10056,#10057,#5392,.T.);
#12395=EDGE_CURVE('',#10057,#10057,#9053,.T.);
#12396=EDGE_CURVE('',#10058,#10058,#9054,.T.);
#12397=EDGE_CURVE('',#10059,#10059,#9055,.T.);
#12398=EDGE_CURVE('',#10060,#10060,#9056,.T.);
#12399=EDGE_CURVE('',#10061,#10061,#9057,.T.);
#12400=EDGE_CURVE('',#10048,#10062,#5393,.T.);
#12401=EDGE_CURVE('',#10062,#10063,#9058,.T.);
#12402=EDGE_CURVE('',#10063,#10062,#9059,.T.);
#12403=EDGE_CURVE('',#10064,#10064,#9060,.T.);
#12404=EDGE_CURVE('',#10064,#10063,#5394,.T.);
#12405=EDGE_CURVE('',#10043,#10065,#5395,.T.);
#12406=EDGE_CURVE('',#10065,#10066,#9061,.T.);
#12407=EDGE_CURVE('',#10066,#10065,#9062,.T.);
#12408=EDGE_CURVE('',#10067,#10067,#9063,.T.);
#12409=EDGE_CURVE('',#10067,#10066,#5396,.T.);
#12410=EDGE_CURVE('',#10047,#10068,#5397,.T.);
#12411=EDGE_CURVE('',#10068,#10069,#9064,.T.);
#12412=EDGE_CURVE('',#10069,#10068,#9065,.T.);
#12413=EDGE_CURVE('',#10070,#10070,#9066,.T.);
#12414=EDGE_CURVE('',#10070,#10069,#5398,.T.);
#12415=EDGE_CURVE('',#10044,#10071,#5399,.T.);
#12416=EDGE_CURVE('',#10071,#10072,#9067,.T.);
#12417=EDGE_CURVE('',#10072,#10071,#9068,.T.);
#12418=EDGE_CURVE('',#10073,#10073,#9069,.T.);
#12419=EDGE_CURVE('',#10073,#10072,#5400,.T.);
#12420=EDGE_CURVE('',#10046,#10074,#5401,.T.);
#12421=EDGE_CURVE('',#10074,#10075,#9070,.T.);
#12422=EDGE_CURVE('',#10075,#10074,#9071,.T.);
#12423=EDGE_CURVE('',#10076,#10076,#9072,.T.);
#12424=EDGE_CURVE('',#10076,#10075,#5402,.T.);
#12425=EDGE_CURVE('',#10045,#10077,#5403,.T.);
#12426=EDGE_CURVE('',#10077,#10078,#9073,.T.);
#12427=EDGE_CURVE('',#10078,#10077,#9074,.T.);
#12428=EDGE_CURVE('',#10079,#10079,#9075,.T.);
#12429=EDGE_CURVE('',#10079,#10078,#5404,.T.);
#12430=EDGE_CURVE('',#10033,#10080,#5405,.T.);
#12431=EDGE_CURVE('',#10080,#10081,#9076,.T.);
#12432=EDGE_CURVE('',#10081,#10080,#9077,.T.);
#12433=EDGE_CURVE('',#10081,#10082,#5406,.T.);
#12434=EDGE_CURVE('',#10082,#10082,#9078,.T.);
#12435=EDGE_CURVE('',#10082,#10083,#5407,.T.);
#12436=EDGE_CURVE('',#10083,#10083,#9079,.T.);
#12437=EDGE_CURVE('',#10084,#10084,#9080,.T.);
#12438=EDGE_CURVE('',#10030,#10085,#5408,.T.);
#12439=EDGE_CURVE('',#10085,#10085,#9081,.T.);
#12440=EDGE_CURVE('',#10086,#10086,#9082,.T.);
#12441=EDGE_CURVE('',#10086,#10084,#5409,.T.);
#12442=EDGE_CURVE('',#10087,#10088,#5410,.T.);
#12443=EDGE_CURVE('',#10088,#10088,#9083,.T.);
#12444=EDGE_CURVE('',#10088,#10089,#5411,.T.);
#12445=EDGE_CURVE('',#10089,#10089,#9084,.T.);
#12446=EDGE_CURVE('',#10089,#10061,#5412,.T.);
#12447=EDGE_CURVE('',#10090,#10091,#5413,.T.);
#12448=EDGE_CURVE('',#10091,#10091,#9085,.T.);
#12449=EDGE_CURVE('',#10091,#10092,#5414,.T.);
#12450=EDGE_CURVE('',#10092,#10092,#9086,.T.);
#12451=EDGE_CURVE('',#10092,#10060,#5415,.T.);
#12452=EDGE_CURVE('',#10093,#10094,#5416,.T.);
#12453=EDGE_CURVE('',#10094,#10094,#9087,.T.);
#12454=EDGE_CURVE('',#10094,#10095,#5417,.T.);
#12455=EDGE_CURVE('',#10095,#10095,#9088,.T.);
#12456=EDGE_CURVE('',#10095,#10059,#5418,.T.);
#12457=EDGE_CURVE('',#10040,#10096,#5419,.T.);
#12458=EDGE_CURVE('',#10096,#10096,#9089,.T.);
#12459=EDGE_CURVE('',#10096,#10097,#5420,.T.);
#12460=EDGE_CURVE('',#10097,#10097,#9090,.T.);
#12461=EDGE_CURVE('',#10097,#10098,#5421,.T.);
#12462=EDGE_CURVE('',#10098,#10098,#9091,.T.);
#12463=EDGE_CURVE('',#10039,#10099,#5422,.T.);
#12464=EDGE_CURVE('',#10099,#10099,#9092,.T.);
#12465=EDGE_CURVE('',#10099,#10100,#5423,.T.);
#12466=EDGE_CURVE('',#10100,#10100,#9093,.T.);
#12467=EDGE_CURVE('',#10100,#10101,#5424,.T.);
#12468=EDGE_CURVE('',#10101,#10101,#9094,.T.);
#12469=EDGE_CURVE('',#10038,#10102,#5425,.T.);
#12470=EDGE_CURVE('',#10102,#10102,#9095,.T.);
#12471=EDGE_CURVE('',#10102,#10103,#5426,.T.);
#12472=EDGE_CURVE('',#10103,#10103,#9096,.T.);
#12473=EDGE_CURVE('',#10103,#10104,#5427,.T.);
#12474=EDGE_CURVE('',#10104,#10104,#9097,.T.);
#12475=EDGE_CURVE('',#10037,#10105,#5428,.T.);
#12476=EDGE_CURVE('',#10105,#10105,#9098,.T.);
#12477=EDGE_CURVE('',#10105,#10106,#5429,.T.);
#12478=EDGE_CURVE('',#10106,#10106,#9099,.T.);
#12479=EDGE_CURVE('',#10106,#10107,#5430,.T.);
#12480=EDGE_CURVE('',#10107,#10107,#9100,.T.);
#12481=EDGE_CURVE('',#10036,#10108,#5431,.T.);
#12482=EDGE_CURVE('',#10108,#10108,#9101,.T.);
#12483=EDGE_CURVE('',#10108,#10109,#5432,.T.);
#12484=EDGE_CURVE('',#10109,#10109,#9102,.T.);
#12485=EDGE_CURVE('',#10109,#10110,#5433,.T.);
#12486=EDGE_CURVE('',#10110,#10110,#9103,.T.);
#12487=EDGE_CURVE('',#10035,#10111,#5434,.T.);
#12488=EDGE_CURVE('',#10111,#10111,#9104,.T.);
#12489=EDGE_CURVE('',#10111,#10112,#5435,.T.);
#12490=EDGE_CURVE('',#10112,#10112,#9105,.T.);
#12491=EDGE_CURVE('',#10112,#10113,#5436,.T.);
#12492=EDGE_CURVE('',#10113,#10113,#9106,.T.);
#12493=EDGE_CURVE('',#10058,#10114,#5437,.T.);
#12494=EDGE_CURVE('',#10114,#10115,#9107,.T.);
#12495=EDGE_CURVE('',#10115,#10114,#9108,.T.);
#12496=EDGE_CURVE('',#10115,#10034,#5438,.T.);
#15886=ORIENTED_EDGE('',*,*,#12351,.T.);
#15887=ORIENTED_EDGE('',*,*,#12352,.T.);
#15888=ORIENTED_EDGE('',*,*,#12353,.T.);
#15889=ORIENTED_EDGE('',*,*,#12354,.T.);
#15890=ORIENTED_EDGE('',*,*,#12352,.F.);
#15891=ORIENTED_EDGE('',*,*,#12351,.F.);
#15892=ORIENTED_EDGE('',*,*,#12355,.T.);
#15893=ORIENTED_EDGE('',*,*,#12356,.F.);
#15894=ORIENTED_EDGE('',*,*,#12355,.F.);
#15895=ORIENTED_EDGE('',*,*,#12357,.F.);
#15896=ORIENTED_EDGE('',*,*,#12358,.T.);
#15897=ORIENTED_EDGE('',*,*,#12353,.F.);
#15898=ORIENTED_EDGE('',*,*,#12354,.F.);
#15899=ORIENTED_EDGE('',*,*,#12358,.F.);
#15900=ORIENTED_EDGE('',*,*,#12359,.T.);
#15901=ORIENTED_EDGE('',*,*,#12360,.T.);
#15902=ORIENTED_EDGE('',*,*,#12361,.T.);
#15903=ORIENTED_EDGE('',*,*,#12360,.F.);
#15904=ORIENTED_EDGE('',*,*,#12359,.F.);
#15905=ORIENTED_EDGE('',*,*,#12362,.T.);
#15906=ORIENTED_EDGE('',*,*,#12363,.F.);
#15907=ORIENTED_EDGE('',*,*,#12362,.F.);
#15908=ORIENTED_EDGE('',*,*,#12361,.F.);
#15909=ORIENTED_EDGE('',*,*,#12364,.F.);
#15910=ORIENTED_EDGE('',*,*,#12365,.T.);
#15911=ORIENTED_EDGE('',*,*,#12366,.T.);
#15912=ORIENTED_EDGE('',*,*,#12367,.T.);
#15913=ORIENTED_EDGE('',*,*,#12368,.T.);
#15914=ORIENTED_EDGE('',*,*,#12369,.T.);
#15915=ORIENTED_EDGE('',*,*,#12370,.T.);
#15916=ORIENTED_EDGE('',*,*,#12356,.T.);
#15917=ORIENTED_EDGE('',*,*,#12371,.T.);
#15918=ORIENTED_EDGE('',*,*,#12372,.T.);
#15919=ORIENTED_EDGE('',*,*,#12371,.F.);
#15920=ORIENTED_EDGE('',*,*,#12372,.F.);
#15921=ORIENTED_EDGE('',*,*,#12373,.F.);
#15922=ORIENTED_EDGE('',*,*,#12374,.F.);
#15923=ORIENTED_EDGE('',*,*,#12375,.F.);
#15924=ORIENTED_EDGE('',*,*,#12376,.F.);
#15925=ORIENTED_EDGE('',*,*,#12377,.F.);
#15926=ORIENTED_EDGE('',*,*,#12378,.F.);
#15927=ORIENTED_EDGE('',*,*,#12379,.F.);
#15928=ORIENTED_EDGE('',*,*,#12380,.T.);
#15929=ORIENTED_EDGE('',*,*,#12381,.T.);
#15930=ORIENTED_EDGE('',*,*,#12373,.T.);
#15931=ORIENTED_EDGE('',*,*,#12381,.F.);
#15932=ORIENTED_EDGE('',*,*,#12380,.F.);
#15933=ORIENTED_EDGE('',*,*,#12382,.T.);
#15934=ORIENTED_EDGE('',*,*,#12383,.F.);
#15935=ORIENTED_EDGE('',*,*,#12382,.F.);
#15936=ORIENTED_EDGE('',*,*,#12383,.T.);
#15937=ORIENTED_EDGE('',*,*,#12384,.T.);
#15938=ORIENTED_EDGE('',*,*,#12385,.T.);
#15939=ORIENTED_EDGE('',*,*,#12386,.T.);
#15940=ORIENTED_EDGE('',*,*,#12384,.F.);
#15941=ORIENTED_EDGE('',*,*,#12387,.F.);
#15942=ORIENTED_EDGE('',*,*,#12388,.F.);
#15943=ORIENTED_EDGE('',*,*,#12389,.T.);
#15944=ORIENTED_EDGE('',*,*,#12385,.F.);
#15945=ORIENTED_EDGE('',*,*,#12386,.F.);
#15946=ORIENTED_EDGE('',*,*,#12389,.F.);
#15947=ORIENTED_EDGE('',*,*,#12390,.T.);
#15948=ORIENTED_EDGE('',*,*,#12391,.T.);
#15949=ORIENTED_EDGE('',*,*,#12387,.T.);
#15950=ORIENTED_EDGE('',*,*,#12388,.T.);
#15951=ORIENTED_EDGE('',*,*,#12391,.F.);
#15952=ORIENTED_EDGE('',*,*,#12390,.F.);
#15953=ORIENTED_EDGE('',*,*,#12392,.T.);
#15954=ORIENTED_EDGE('',*,*,#12393,.F.);
#15955=ORIENTED_EDGE('',*,*,#12392,.F.);
#15956=ORIENTED_EDGE('',*,*,#12393,.T.);
#15957=ORIENTED_EDGE('',*,*,#12394,.T.);
#15958=ORIENTED_EDGE('',*,*,#12395,.T.);
#15959=ORIENTED_EDGE('',*,*,#12394,.F.);
#15960=ORIENTED_EDGE('',*,*,#12396,.F.);
#15961=ORIENTED_EDGE('',*,*,#12397,.T.);
#15962=ORIENTED_EDGE('',*,*,#12398,.T.);
#15963=ORIENTED_EDGE('',*,*,#12399,.T.);
#15964=ORIENTED_EDGE('',*,*,#12395,.F.);
#15965=ORIENTED_EDGE('',*,*,#12379,.T.);
#15966=ORIENTED_EDGE('',*,*,#12400,.T.);
#15967=ORIENTED_EDGE('',*,*,#12401,.T.);
#15968=ORIENTED_EDGE('',*,*,#12402,.T.);
#15969=ORIENTED_EDGE('',*,*,#12400,.F.);
#15970=ORIENTED_EDGE('',*,*,#12403,.F.);
#15971=ORIENTED_EDGE('',*,*,#12404,.T.);
#15972=ORIENTED_EDGE('',*,*,#12401,.F.);
#15973=ORIENTED_EDGE('',*,*,#12402,.F.);
#15974=ORIENTED_EDGE('',*,*,#12404,.F.);
#15975=ORIENTED_EDGE('',*,*,#12374,.T.);
#15976=ORIENTED_EDGE('',*,*,#12405,.T.);
#15977=ORIENTED_EDGE('',*,*,#12406,.T.);
#15978=ORIENTED_EDGE('',*,*,#12407,.T.);
#15979=ORIENTED_EDGE('',*,*,#12405,.F.);
#15980=ORIENTED_EDGE('',*,*,#12408,.F.);
#15981=ORIENTED_EDGE('',*,*,#12409,.T.);
#15982=ORIENTED_EDGE('',*,*,#12406,.F.);
#15983=ORIENTED_EDGE('',*,*,#12407,.F.);
#15984=ORIENTED_EDGE('',*,*,#12409,.F.);
#15985=ORIENTED_EDGE('',*,*,#12378,.T.);
#15986=ORIENTED_EDGE('',*,*,#12410,.T.);
#15987=ORIENTED_EDGE('',*,*,#12411,.T.);
#15988=ORIENTED_EDGE('',*,*,#12412,.T.);
#15989=ORIENTED_EDGE('',*,*,#12410,.F.);
#15990=ORIENTED_EDGE('',*,*,#12413,.F.);
#15991=ORIENTED_EDGE('',*,*,#12414,.T.);
#15992=ORIENTED_EDGE('',*,*,#12411,.F.);
#15993=ORIENTED_EDGE('',*,*,#12412,.F.);
#15994=ORIENTED_EDGE('',*,*,#12414,.F.);
#15995=ORIENTED_EDGE('',*,*,#12375,.T.);
#15996=ORIENTED_EDGE('',*,*,#12415,.T.);
#15997=ORIENTED_EDGE('',*,*,#12416,.T.);
#15998=ORIENTED_EDGE('',*,*,#12417,.T.);
#15999=ORIENTED_EDGE('',*,*,#12415,.F.);
#16000=ORIENTED_EDGE('',*,*,#12418,.F.);
#16001=ORIENTED_EDGE('',*,*,#12419,.T.);
#16002=ORIENTED_EDGE('',*,*,#12416,.F.);
#16003=ORIENTED_EDGE('',*,*,#12417,.F.);
#16004=ORIENTED_EDGE('',*,*,#12419,.F.);
#16005=ORIENTED_EDGE('',*,*,#12377,.T.);
#16006=ORIENTED_EDGE('',*,*,#12420,.T.);
#16007=ORIENTED_EDGE('',*,*,#12421,.T.);
#16008=ORIENTED_EDGE('',*,*,#12422,.T.);
#16009=ORIENTED_EDGE('',*,*,#12420,.F.);
#16010=ORIENTED_EDGE('',*,*,#12423,.F.);
#16011=ORIENTED_EDGE('',*,*,#12424,.T.);
#16012=ORIENTED_EDGE('',*,*,#12421,.F.);
#16013=ORIENTED_EDGE('',*,*,#12422,.F.);
#16014=ORIENTED_EDGE('',*,*,#12424,.F.);
#16015=ORIENTED_EDGE('',*,*,#12376,.T.);
#16016=ORIENTED_EDGE('',*,*,#12425,.T.);
#16017=ORIENTED_EDGE('',*,*,#12426,.T.);
#16018=ORIENTED_EDGE('',*,*,#12427,.T.);
#16019=ORIENTED_EDGE('',*,*,#12425,.F.);
#16020=ORIENTED_EDGE('',*,*,#12428,.F.);
#16021=ORIENTED_EDGE('',*,*,#12429,.T.);
#16022=ORIENTED_EDGE('',*,*,#12426,.F.);
#16023=ORIENTED_EDGE('',*,*,#12427,.F.);
#16024=ORIENTED_EDGE('',*,*,#12429,.F.);
#16025=ORIENTED_EDGE('',*,*,#12363,.T.);
#16026=ORIENTED_EDGE('',*,*,#12430,.T.);
#16027=ORIENTED_EDGE('',*,*,#12431,.T.);
#16028=ORIENTED_EDGE('',*,*,#12432,.T.);
#16029=ORIENTED_EDGE('',*,*,#12430,.F.);
#16030=ORIENTED_EDGE('',*,*,#12431,.F.);
#16031=ORIENTED_EDGE('',*,*,#12432,.F.);
#16032=ORIENTED_EDGE('',*,*,#12433,.T.);
#16033=ORIENTED_EDGE('',*,*,#12434,.F.);
#16034=ORIENTED_EDGE('',*,*,#12433,.F.);
#16035=ORIENTED_EDGE('',*,*,#12434,.T.);
#16036=ORIENTED_EDGE('',*,*,#12435,.T.);
#16037=ORIENTED_EDGE('',*,*,#12436,.T.);
#16038=ORIENTED_EDGE('',*,*,#12435,.F.);
#16039=ORIENTED_EDGE('',*,*,#12436,.F.);
#16040=ORIENTED_EDGE('',*,*,#12437,.T.);
#16041=ORIENTED_EDGE('',*,*,#12357,.T.);
#16042=ORIENTED_EDGE('',*,*,#12438,.T.);
#16043=ORIENTED_EDGE('',*,*,#12439,.T.);
#16044=ORIENTED_EDGE('',*,*,#12438,.F.);
#16045=ORIENTED_EDGE('',*,*,#12439,.F.);
#16046=ORIENTED_EDGE('',*,*,#12440,.F.);
#16047=ORIENTED_EDGE('',*,*,#12440,.T.);
#16048=ORIENTED_EDGE('',*,*,#12441,.T.);
#16049=ORIENTED_EDGE('',*,*,#12437,.F.);
#16050=ORIENTED_EDGE('',*,*,#12441,.F.);
#16051=ORIENTED_EDGE('',*,*,#12442,.T.);
#16052=ORIENTED_EDGE('',*,*,#12443,.T.);
#16053=ORIENTED_EDGE('',*,*,#12442,.F.);
#16054=ORIENTED_EDGE('',*,*,#12443,.F.);
#16055=ORIENTED_EDGE('',*,*,#12444,.T.);
#16056=ORIENTED_EDGE('',*,*,#12445,.T.);
#16057=ORIENTED_EDGE('',*,*,#12444,.F.);
#16058=ORIENTED_EDGE('',*,*,#12445,.F.);
#16059=ORIENTED_EDGE('',*,*,#12446,.T.);
#16060=ORIENTED_EDGE('',*,*,#12399,.F.);
#16061=ORIENTED_EDGE('',*,*,#12446,.F.);
#16062=ORIENTED_EDGE('',*,*,#12447,.T.);
#16063=ORIENTED_EDGE('',*,*,#12448,.T.);
#16064=ORIENTED_EDGE('',*,*,#12447,.F.);
#16065=ORIENTED_EDGE('',*,*,#12448,.F.);
#16066=ORIENTED_EDGE('',*,*,#12449,.T.);
#16067=ORIENTED_EDGE('',*,*,#12450,.T.);
#16068=ORIENTED_EDGE('',*,*,#12449,.F.);
#16069=ORIENTED_EDGE('',*,*,#12450,.F.);
#16070=ORIENTED_EDGE('',*,*,#12451,.T.);
#16071=ORIENTED_EDGE('',*,*,#12398,.F.);
#16072=ORIENTED_EDGE('',*,*,#12451,.F.);
#16073=ORIENTED_EDGE('',*,*,#12452,.T.);
#16074=ORIENTED_EDGE('',*,*,#12453,.T.);
#16075=ORIENTED_EDGE('',*,*,#12452,.F.);
#16076=ORIENTED_EDGE('',*,*,#12453,.F.);
#16077=ORIENTED_EDGE('',*,*,#12454,.T.);
#16078=ORIENTED_EDGE('',*,*,#12455,.T.);
#16079=ORIENTED_EDGE('',*,*,#12454,.F.);
#16080=ORIENTED_EDGE('',*,*,#12455,.F.);
#16081=ORIENTED_EDGE('',*,*,#12456,.T.);
#16082=ORIENTED_EDGE('',*,*,#12397,.F.);
#16083=ORIENTED_EDGE('',*,*,#12456,.F.);
#16084=ORIENTED_EDGE('',*,*,#12370,.F.);
#16085=ORIENTED_EDGE('',*,*,#12457,.T.);
#16086=ORIENTED_EDGE('',*,*,#12458,.T.);
#16087=ORIENTED_EDGE('',*,*,#12457,.F.);
#16088=ORIENTED_EDGE('',*,*,#12458,.F.);
#16089=ORIENTED_EDGE('',*,*,#12459,.T.);
#16090=ORIENTED_EDGE('',*,*,#12460,.T.);
#16091=ORIENTED_EDGE('',*,*,#12459,.F.);
#16092=ORIENTED_EDGE('',*,*,#12460,.F.);
#16093=ORIENTED_EDGE('',*,*,#12461,.T.);
#16094=ORIENTED_EDGE('',*,*,#12462,.T.);
#16095=ORIENTED_EDGE('',*,*,#12461,.F.);
#16096=ORIENTED_EDGE('',*,*,#12428,.T.);
#16097=ORIENTED_EDGE('',*,*,#12462,.F.);
#16098=ORIENTED_EDGE('',*,*,#12369,.F.);
#16099=ORIENTED_EDGE('',*,*,#12463,.T.);
#16100=ORIENTED_EDGE('',*,*,#12464,.T.);
#16101=ORIENTED_EDGE('',*,*,#12463,.F.);
#16102=ORIENTED_EDGE('',*,*,#12464,.F.);
#16103=ORIENTED_EDGE('',*,*,#12465,.T.);
#16104=ORIENTED_EDGE('',*,*,#12466,.T.);
#16105=ORIENTED_EDGE('',*,*,#12465,.F.);
#16106=ORIENTED_EDGE('',*,*,#12466,.F.);
#16107=ORIENTED_EDGE('',*,*,#12467,.T.);
#16108=ORIENTED_EDGE('',*,*,#12468,.T.);
#16109=ORIENTED_EDGE('',*,*,#12467,.F.);
#16110=ORIENTED_EDGE('',*,*,#12423,.T.);
#16111=ORIENTED_EDGE('',*,*,#12468,.F.);
#16112=ORIENTED_EDGE('',*,*,#12368,.F.);
#16113=ORIENTED_EDGE('',*,*,#12469,.T.);
#16114=ORIENTED_EDGE('',*,*,#12470,.T.);
#16115=ORIENTED_EDGE('',*,*,#12469,.F.);
#16116=ORIENTED_EDGE('',*,*,#12470,.F.);
#16117=ORIENTED_EDGE('',*,*,#12471,.T.);
#16118=ORIENTED_EDGE('',*,*,#12472,.T.);
#16119=ORIENTED_EDGE('',*,*,#12471,.F.);
#16120=ORIENTED_EDGE('',*,*,#12472,.F.);
#16121=ORIENTED_EDGE('',*,*,#12473,.T.);
#16122=ORIENTED_EDGE('',*,*,#12474,.T.);
#16123=ORIENTED_EDGE('',*,*,#12473,.F.);
#16124=ORIENTED_EDGE('',*,*,#12418,.T.);
#16125=ORIENTED_EDGE('',*,*,#12474,.F.);
#16126=ORIENTED_EDGE('',*,*,#12367,.F.);
#16127=ORIENTED_EDGE('',*,*,#12475,.T.);
#16128=ORIENTED_EDGE('',*,*,#12476,.T.);
#16129=ORIENTED_EDGE('',*,*,#12475,.F.);
#16130=ORIENTED_EDGE('',*,*,#12476,.F.);
#16131=ORIENTED_EDGE('',*,*,#12477,.T.);
#16132=ORIENTED_EDGE('',*,*,#12478,.T.);
#16133=ORIENTED_EDGE('',*,*,#12477,.F.);
#16134=ORIENTED_EDGE('',*,*,#12478,.F.);
#16135=ORIENTED_EDGE('',*,*,#12479,.T.);
#16136=ORIENTED_EDGE('',*,*,#12480,.T.);
#16137=ORIENTED_EDGE('',*,*,#12479,.F.);
#16138=ORIENTED_EDGE('',*,*,#12413,.T.);
#16139=ORIENTED_EDGE('',*,*,#12480,.F.);
#16140=ORIENTED_EDGE('',*,*,#12366,.F.);
#16141=ORIENTED_EDGE('',*,*,#12481,.T.);
#16142=ORIENTED_EDGE('',*,*,#12482,.T.);
#16143=ORIENTED_EDGE('',*,*,#12481,.F.);
#16144=ORIENTED_EDGE('',*,*,#12482,.F.);
#16145=ORIENTED_EDGE('',*,*,#12483,.T.);
#16146=ORIENTED_EDGE('',*,*,#12484,.T.);
#16147=ORIENTED_EDGE('',*,*,#12483,.F.);
#16148=ORIENTED_EDGE('',*,*,#12484,.F.);
#16149=ORIENTED_EDGE('',*,*,#12485,.T.);
#16150=ORIENTED_EDGE('',*,*,#12486,.T.);
#16151=ORIENTED_EDGE('',*,*,#12485,.F.);
#16152=ORIENTED_EDGE('',*,*,#12408,.T.);
#16153=ORIENTED_EDGE('',*,*,#12486,.F.);
#16154=ORIENTED_EDGE('',*,*,#12365,.F.);
#16155=ORIENTED_EDGE('',*,*,#12487,.T.);
#16156=ORIENTED_EDGE('',*,*,#12488,.T.);
#16157=ORIENTED_EDGE('',*,*,#12487,.F.);
#16158=ORIENTED_EDGE('',*,*,#12488,.F.);
#16159=ORIENTED_EDGE('',*,*,#12489,.T.);
#16160=ORIENTED_EDGE('',*,*,#12490,.T.);
#16161=ORIENTED_EDGE('',*,*,#12489,.F.);
#16162=ORIENTED_EDGE('',*,*,#12490,.F.);
#16163=ORIENTED_EDGE('',*,*,#12491,.T.);
#16164=ORIENTED_EDGE('',*,*,#12492,.T.);
#16165=ORIENTED_EDGE('',*,*,#12491,.F.);
#16166=ORIENTED_EDGE('',*,*,#12403,.T.);
#16167=ORIENTED_EDGE('',*,*,#12492,.F.);
#16168=ORIENTED_EDGE('',*,*,#12396,.T.);
#16169=ORIENTED_EDGE('',*,*,#12493,.T.);
#16170=ORIENTED_EDGE('',*,*,#12494,.T.);
#16171=ORIENTED_EDGE('',*,*,#12495,.T.);
#16172=ORIENTED_EDGE('',*,*,#12493,.F.);
#16173=ORIENTED_EDGE('',*,*,#12494,.F.);
#16174=ORIENTED_EDGE('',*,*,#12495,.F.);
#16175=ORIENTED_EDGE('',*,*,#12496,.T.);
#16176=ORIENTED_EDGE('',*,*,#12364,.T.);
#16177=ORIENTED_EDGE('',*,*,#12496,.F.);
#22956=CONICAL_SURFACE('',#24772,4.7393933982822,0.392699081698728);
#22957=CONICAL_SURFACE('',#24776,4.71,0.785398163397448);
#22958=CONICAL_SURFACE('',#24780,4.6656066017178,1.17809724509617);
#22959=CONICAL_SURFACE('',#24783,4.71,0.785398163397448);
#22960=CONICAL_SURFACE('',#24793,4.6656066017178,1.17809724509617);
#22961=CONICAL_SURFACE('',#24803,0.754393398282202,1.17809724509617);
#22962=CONICAL_SURFACE('',#24805,0.725,0.785398163397448);
#22963=CONICAL_SURFACE('',#24807,0.710606601717798,0.392699081698724);
#22964=CONICAL_SURFACE('',#24813,0.710606601717798,0.392699081698723);
#22965=CONICAL_SURFACE('',#24815,0.725,0.785398163397448);
#22966=CONICAL_SURFACE('',#24817,0.754393398282202,1.17809724509618);
#22967=CONICAL_SURFACE('',#24824,0.225,0.785398163397452);
#22968=CONICAL_SURFACE('',#24829,0.225,0.785398163397445);
#22969=CONICAL_SURFACE('',#24834,0.225,0.785398163397449);
#22970=CONICAL_SURFACE('',#24839,0.225,0.785398163397452);
#22971=CONICAL_SURFACE('',#24844,0.225,0.785398163397449);
#22972=CONICAL_SURFACE('',#24849,0.225,0.785398163397445);
#22973=CONICAL_SURFACE('',#24854,4.7393933982822,0.392699081698727);
#22974=CONICAL_SURFACE('',#24859,4.735,0.785398163397452);
#22975=CONICAL_SURFACE('',#24863,4.735,0.785398163397452);
#22976=CONICAL_SURFACE('',#24868,0.0649999999999999,1.02974425867665);
#22977=CONICAL_SURFACE('',#24872,0.18,0.78539816339745);
#22978=CONICAL_SURFACE('',#24873,0.0649999999999999,1.02974425867665);
#22979=CONICAL_SURFACE('',#24877,0.18,0.78539816339745);
#22980=CONICAL_SURFACE('',#24878,0.065,1.02974425867665);
#22981=CONICAL_SURFACE('',#24882,0.18,0.785398163397449);
#22982=CONICAL_SURFACE('',#24883,0.1325,0.321750554396641);
#22983=CONICAL_SURFACE('',#24887,0.1325,0.785398163397446);
#22984=CONICAL_SURFACE('',#24890,0.1325,0.321750554396641);
#22985=CONICAL_SURFACE('',#24894,0.1325,0.785398163397446);
#22986=CONICAL_SURFACE('',#24897,0.1325,0.321750554396647);
#22987=CONICAL_SURFACE('',#24901,0.1325,0.785398163397455);
#22988=CONICAL_SURFACE('',#24904,0.132499999999999,0.321750554396641);
#22989=CONICAL_SURFACE('',#24908,0.132499999999999,0.785398163397446);
#22990=CONICAL_SURFACE('',#24911,0.1325,0.321750554396641);
#22991=CONICAL_SURFACE('',#24915,0.1325,0.785398163397446);
#22992=CONICAL_SURFACE('',#24918,0.1325,0.321750554396647);
#22993=CONICAL_SURFACE('',#24922,0.1325,0.785398163397455);
#22994=CONICAL_SURFACE('',#24925,4.075,0.785398163397448);
#23165=ADVANCED_FACE('',(#2412),#22956,.T.);
#23166=ADVANCED_FACE('',(#2413),#22957,.T.);
#23167=ADVANCED_FACE('',(#2414),#1952,.T.);
#23168=ADVANCED_FACE('',(#2415),#22958,.T.);
#23169=ADVANCED_FACE('',(#2416),#22959,.T.);
#23170=ADVANCED_FACE('',(#2417,#1036,#1037,#1038,#1039,#1040,#1041,#1042),
#1276,.T.);
#23171=ADVANCED_FACE('',(#2418),#22960,.T.);
#23172=ADVANCED_FACE('',(#2419,#1043,#1044,#1045,#1046,#1047,#1048,#1049),
#1277,.T.);
#23173=ADVANCED_FACE('',(#2420),#22961,.F.);
#23174=ADVANCED_FACE('',(#2421),#22962,.F.);
#23175=ADVANCED_FACE('',(#2422),#22963,.F.);
#23176=ADVANCED_FACE('',(#2423),#1953,.F.);
#23177=ADVANCED_FACE('',(#2424),#22964,.F.);
#23178=ADVANCED_FACE('',(#2425),#22965,.F.);
#23179=ADVANCED_FACE('',(#2426),#22966,.F.);
#23180=ADVANCED_FACE('',(#2427,#1050,#1051,#1052,#1053),#1278,.T.);
#23181=ADVANCED_FACE('',(#2428),#22967,.F.);
#23182=ADVANCED_FACE('',(#2429),#1954,.F.);
#23183=ADVANCED_FACE('',(#2430),#22968,.F.);
#23184=ADVANCED_FACE('',(#2431),#1955,.F.);
#23185=ADVANCED_FACE('',(#2432),#22969,.F.);
#23186=ADVANCED_FACE('',(#2433),#1956,.F.);
#23187=ADVANCED_FACE('',(#2434),#22970,.F.);
#23188=ADVANCED_FACE('',(#2435),#1957,.F.);
#23189=ADVANCED_FACE('',(#2436),#22971,.F.);
#23190=ADVANCED_FACE('',(#2437),#1958,.F.);
#23191=ADVANCED_FACE('',(#2438),#22972,.F.);
#23192=ADVANCED_FACE('',(#2439),#1959,.F.);
#23193=ADVANCED_FACE('',(#2440),#22973,.T.);
#23194=ADVANCED_FACE('',(#2441),#1960,.T.);
#23195=ADVANCED_FACE('',(#2442),#22974,.T.);
#23196=ADVANCED_FACE('',(#2443,#1054),#1279,.F.);
#23197=ADVANCED_FACE('',(#2444),#22975,.T.);
#23198=ADVANCED_FACE('',(#2445,#1055),#1280,.F.);
#23199=ADVANCED_FACE('',(#2446),#1961,.T.);
#23200=ADVANCED_FACE('',(#2447),#22976,.F.);
#23201=ADVANCED_FACE('',(#2448),#1962,.F.);
#23202=ADVANCED_FACE('',(#2449),#22977,.F.);
#23203=ADVANCED_FACE('',(#2450),#22978,.F.);
#23204=ADVANCED_FACE('',(#2451),#1963,.F.);
#23205=ADVANCED_FACE('',(#2452),#22979,.F.);
#23206=ADVANCED_FACE('',(#2453),#22980,.F.);
#23207=ADVANCED_FACE('',(#2454),#1964,.F.);
#23208=ADVANCED_FACE('',(#2455),#22981,.F.);
#23209=ADVANCED_FACE('',(#2456),#22982,.F.);
#23210=ADVANCED_FACE('',(#2457),#1965,.F.);
#23211=ADVANCED_FACE('',(#2458),#22983,.F.);
#23212=ADVANCED_FACE('',(#2459,#1056),#1281,.F.);
#23213=ADVANCED_FACE('',(#2460),#22984,.F.);
#23214=ADVANCED_FACE('',(#2461),#1966,.F.);
#23215=ADVANCED_FACE('',(#2462),#22985,.F.);
#23216=ADVANCED_FACE('',(#2463,#1057),#1282,.F.);
#23217=ADVANCED_FACE('',(#2464),#22986,.F.);
#23218=ADVANCED_FACE('',(#2465),#1967,.F.);
#23219=ADVANCED_FACE('',(#2466),#22987,.F.);
#23220=ADVANCED_FACE('',(#2467,#1058),#1283,.F.);
#23221=ADVANCED_FACE('',(#2468),#22988,.F.);
#23222=ADVANCED_FACE('',(#2469),#1968,.F.);
#23223=ADVANCED_FACE('',(#2470),#22989,.F.);
#23224=ADVANCED_FACE('',(#2471,#1059),#1284,.F.);
#23225=ADVANCED_FACE('',(#2472),#22990,.F.);
#23226=ADVANCED_FACE('',(#2473),#1969,.F.);
#23227=ADVANCED_FACE('',(#2474),#22991,.F.);
#23228=ADVANCED_FACE('',(#2475,#1060),#1285,.F.);
#23229=ADVANCED_FACE('',(#2476),#22992,.F.);
#23230=ADVANCED_FACE('',(#2477),#1970,.F.);
#23231=ADVANCED_FACE('',(#2478),#22993,.F.);
#23232=ADVANCED_FACE('',(#2479,#1061),#1286,.F.);
#23233=ADVANCED_FACE('',(#2480),#22994,.T.);
#23234=ADVANCED_FACE('',(#2481),#1971,.T.);
#24529=CLOSED_SHELL('',(#23165,#23166,#23167,#23168,#23169,#23170,#23171,
#23172,#23173,#23174,#23175,#23176,#23177,#23178,#23179,#23180,#23181,#23182,
#23183,#23184,#23185,#23186,#23187,#23188,#23189,#23190,#23191,#23192,#23193,
#23194,#23195,#23196,#23197,#23198,#23199,#23200,#23201,#23202,#23203,#23204,
#23205,#23206,#23207,#23208,#23209,#23210,#23211,#23212,#23213,#23214,#23215,
#23216,#23217,#23218,#23219,#23220,#23221,#23222,#23223,#23224,#23225,#23226,
#23227,#23228,#23229,#23230,#23231,#23232,#23233,#23234));
#24771=AXIS2_PLACEMENT_3D('',#33870,#27198,#27199);
#24772=AXIS2_PLACEMENT_3D('',#33871,#27200,#27201);
#24773=AXIS2_PLACEMENT_3D('',#33873,#27202,#27203);
#24774=AXIS2_PLACEMENT_3D('',#33877,#27205,#27206);
#24775=AXIS2_PLACEMENT_3D('',#33878,#27207,#27208);
#24776=AXIS2_PLACEMENT_3D('',#33879,#27209,#27210);
#24777=AXIS2_PLACEMENT_3D('',#33882,#27212,#27213);
#24778=AXIS2_PLACEMENT_3D('',#33883,#27214,#27215);
#24779=AXIS2_PLACEMENT_3D('',#33885,#27216,#27217);
#24780=AXIS2_PLACEMENT_3D('',#33887,#27219,#27220);
#24781=AXIS2_PLACEMENT_3D('',#33889,#27221,#27222);
#24782=AXIS2_PLACEMENT_3D('',#33892,#27224,#27225);
#24783=AXIS2_PLACEMENT_3D('',#33893,#27226,#27227);
#24784=AXIS2_PLACEMENT_3D('',#33896,#27229,#27230);
#24785=AXIS2_PLACEMENT_3D('',#33897,#27231,#27232);
#24786=AXIS2_PLACEMENT_3D('',#33899,#27233,#27234);
#24787=AXIS2_PLACEMENT_3D('',#33901,#27235,#27236);
#24788=AXIS2_PLACEMENT_3D('',#33903,#27237,#27238);
#24789=AXIS2_PLACEMENT_3D('',#33905,#27239,#27240);
#24790=AXIS2_PLACEMENT_3D('',#33907,#27241,#27242);
#24791=AXIS2_PLACEMENT_3D('',#33909,#27243,#27244);
#24792=AXIS2_PLACEMENT_3D('',#33911,#27245,#27246);
#24793=AXIS2_PLACEMENT_3D('',#33912,#27247,#27248);
#24794=AXIS2_PLACEMENT_3D('',#33915,#27250,#27251);
#24795=AXIS2_PLACEMENT_3D('',#33916,#27252,#27253);
#24796=AXIS2_PLACEMENT_3D('',#33918,#27254,#27255);
#24797=AXIS2_PLACEMENT_3D('',#33920,#27256,#27257);
#24798=AXIS2_PLACEMENT_3D('',#33922,#27258,#27259);
#24799=AXIS2_PLACEMENT_3D('',#33924,#27260,#27261);
#24800=AXIS2_PLACEMENT_3D('',#33926,#27262,#27263);
#24801=AXIS2_PLACEMENT_3D('',#33928,#27264,#27265);
#24802=AXIS2_PLACEMENT_3D('',#33930,#27266,#27267);
#24803=AXIS2_PLACEMENT_3D('',#33931,#27268,#27269);
#24804=AXIS2_PLACEMENT_3D('',#33933,#27270,#27271);
#24805=AXIS2_PLACEMENT_3D('',#33935,#27273,#27274);
#24806=AXIS2_PLACEMENT_3D('',#33938,#27276,#27277);
#24807=AXIS2_PLACEMENT_3D('',#33939,#27278,#27279);
#24808=AXIS2_PLACEMENT_3D('',#33943,#27281,#27282);
#24809=AXIS2_PLACEMENT_3D('',#33944,#27283,#27284);
#24810=AXIS2_PLACEMENT_3D('',#33945,#27285,#27286);
#24811=AXIS2_PLACEMENT_3D('',#33948,#27287,#27288);
#24812=AXIS2_PLACEMENT_3D('',#33949,#27289,#27290);
#24813=AXIS2_PLACEMENT_3D('',#33951,#27292,#27293);
#24814=AXIS2_PLACEMENT_3D('',#33953,#27294,#27295);
#24815=AXIS2_PLACEMENT_3D('',#33955,#27297,#27298);
#24816=AXIS2_PLACEMENT_3D('',#33958,#27300,#27301);
#24817=AXIS2_PLACEMENT_3D('',#33959,#27302,#27303);
#24818=AXIS2_PLACEMENT_3D('',#33962,#27305,#27306);
#24819=AXIS2_PLACEMENT_3D('',#33963,#27307,#27308);
#24820=AXIS2_PLACEMENT_3D('',#33965,#27309,#27310);
#24821=AXIS2_PLACEMENT_3D('',#33967,#27311,#27312);
#24822=AXIS2_PLACEMENT_3D('',#33969,#27313,#27314);
#24823=AXIS2_PLACEMENT_3D('',#33971,#27315,#27316);
#24824=AXIS2_PLACEMENT_3D('',#33972,#27317,#27318);
#24825=AXIS2_PLACEMENT_3D('',#33976,#27320,#27321);
#24826=AXIS2_PLACEMENT_3D('',#33977,#27322,#27323);
#24827=AXIS2_PLACEMENT_3D('',#33978,#27324,#27325);
#24828=AXIS2_PLACEMENT_3D('',#33980,#27326,#27327);
#24829=AXIS2_PLACEMENT_3D('',#33982,#27329,#27330);
#24830=AXIS2_PLACEMENT_3D('',#33986,#27332,#27333);
#24831=AXIS2_PLACEMENT_3D('',#33987,#27334,#27335);
#24832=AXIS2_PLACEMENT_3D('',#33988,#27336,#27337);
#24833=AXIS2_PLACEMENT_3D('',#33990,#27338,#27339);
#24834=AXIS2_PLACEMENT_3D('',#33992,#27341,#27342);
#24835=AXIS2_PLACEMENT_3D('',#33996,#27344,#27345);
#24836=AXIS2_PLACEMENT_3D('',#33997,#27346,#27347);
#24837=AXIS2_PLACEMENT_3D('',#33998,#27348,#27349);
#24838=AXIS2_PLACEMENT_3D('',#34000,#27350,#27351);
#24839=AXIS2_PLACEMENT_3D('',#34002,#27353,#27354);
#24840=AXIS2_PLACEMENT_3D('',#34006,#27356,#27357);
#24841=AXIS2_PLACEMENT_3D('',#34007,#27358,#27359);
#24842=AXIS2_PLACEMENT_3D('',#34008,#27360,#27361);
#24843=AXIS2_PLACEMENT_3D('',#34010,#27362,#27363);
#24844=AXIS2_PLACEMENT_3D('',#34012,#27365,#27366);
#24845=AXIS2_PLACEMENT_3D('',#34016,#27368,#27369);
#24846=AXIS2_PLACEMENT_3D('',#34017,#27370,#27371);
#24847=AXIS2_PLACEMENT_3D('',#34018,#27372,#27373);
#24848=AXIS2_PLACEMENT_3D('',#34020,#27374,#27375);
#24849=AXIS2_PLACEMENT_3D('',#34022,#27377,#27378);
#24850=AXIS2_PLACEMENT_3D('',#34026,#27380,#27381);
#24851=AXIS2_PLACEMENT_3D('',#34027,#27382,#27383);
#24852=AXIS2_PLACEMENT_3D('',#34028,#27384,#27385);
#24853=AXIS2_PLACEMENT_3D('',#34030,#27386,#27387);
#24854=AXIS2_PLACEMENT_3D('',#34032,#27389,#27390);
#24855=AXIS2_PLACEMENT_3D('',#34036,#27392,#27393);
#24856=AXIS2_PLACEMENT_3D('',#34037,#27394,#27395);
#24857=AXIS2_PLACEMENT_3D('',#34038,#27396,#27397);
#24858=AXIS2_PLACEMENT_3D('',#34041,#27399,#27400);
#24859=AXIS2_PLACEMENT_3D('',#34042,#27401,#27402);
#24860=AXIS2_PLACEMENT_3D('',#34045,#27404,#27405);
#24861=AXIS2_PLACEMENT_3D('',#34046,#27406,#27407);
#24862=AXIS2_PLACEMENT_3D('',#34048,#27408,#27409);
#24863=AXIS2_PLACEMENT_3D('',#34049,#27410,#27411);
#24864=AXIS2_PLACEMENT_3D('',#34052,#27413,#27414);
#24865=AXIS2_PLACEMENT_3D('',#34053,#27415,#27416);
#24866=AXIS2_PLACEMENT_3D('',#34055,#27417,#27418);
#24867=AXIS2_PLACEMENT_3D('',#34056,#27419,#27420);
#24868=AXIS2_PLACEMENT_3D('',#34058,#27422,#27423);
#24869=AXIS2_PLACEMENT_3D('',#34062,#27425,#27426);
#24870=AXIS2_PLACEMENT_3D('',#34063,#27427,#27428);
#24871=AXIS2_PLACEMENT_3D('',#34066,#27430,#27431);
#24872=AXIS2_PLACEMENT_3D('',#34067,#27432,#27433);
#24873=AXIS2_PLACEMENT_3D('',#34069,#27435,#27436);
#24874=AXIS2_PLACEMENT_3D('',#34073,#27438,#27439);
#24875=AXIS2_PLACEMENT_3D('',#34074,#27440,#27441);
#24876=AXIS2_PLACEMENT_3D('',#34077,#27443,#27444);
#24877=AXIS2_PLACEMENT_3D('',#34078,#27445,#27446);
#24878=AXIS2_PLACEMENT_3D('',#34080,#27448,#27449);
#24879=AXIS2_PLACEMENT_3D('',#34084,#27451,#27452);
#24880=AXIS2_PLACEMENT_3D('',#34085,#27453,#27454);
#24881=AXIS2_PLACEMENT_3D('',#34088,#27456,#27457);
#24882=AXIS2_PLACEMENT_3D('',#34089,#27458,#27459);
#24883=AXIS2_PLACEMENT_3D('',#34091,#27461,#27462);
#24884=AXIS2_PLACEMENT_3D('',#34094,#27464,#27465);
#24885=AXIS2_PLACEMENT_3D('',#34095,#27466,#27467);
#24886=AXIS2_PLACEMENT_3D('',#34098,#27469,#27470);
#24887=AXIS2_PLACEMENT_3D('',#34099,#27471,#27472);
#24888=AXIS2_PLACEMENT_3D('',#34102,#27474,#27475);
#24889=AXIS2_PLACEMENT_3D('',#34103,#27476,#27477);
#24890=AXIS2_PLACEMENT_3D('',#34104,#27478,#27479);
#24891=AXIS2_PLACEMENT_3D('',#34107,#27481,#27482);
#24892=AXIS2_PLACEMENT_3D('',#34108,#27483,#27484);
#24893=AXIS2_PLACEMENT_3D('',#34111,#27486,#27487);
#24894=AXIS2_PLACEMENT_3D('',#34112,#27488,#27489);
#24895=AXIS2_PLACEMENT_3D('',#34115,#27491,#27492);
#24896=AXIS2_PLACEMENT_3D('',#34116,#27493,#27494);
#24897=AXIS2_PLACEMENT_3D('',#34117,#27495,#27496);
#24898=AXIS2_PLACEMENT_3D('',#34120,#27498,#27499);
#24899=AXIS2_PLACEMENT_3D('',#34121,#27500,#27501);
#24900=AXIS2_PLACEMENT_3D('',#34124,#27503,#27504);
#24901=AXIS2_PLACEMENT_3D('',#34125,#27505,#27506);
#24902=AXIS2_PLACEMENT_3D('',#34128,#27508,#27509);
#24903=AXIS2_PLACEMENT_3D('',#34129,#27510,#27511);
#24904=AXIS2_PLACEMENT_3D('',#34130,#27512,#27513);
#24905=AXIS2_PLACEMENT_3D('',#34133,#27515,#27516);
#24906=AXIS2_PLACEMENT_3D('',#34134,#27517,#27518);
#24907=AXIS2_PLACEMENT_3D('',#34137,#27520,#27521);
#24908=AXIS2_PLACEMENT_3D('',#34138,#27522,#27523);
#24909=AXIS2_PLACEMENT_3D('',#34141,#27525,#27526);
#24910=AXIS2_PLACEMENT_3D('',#34142,#27527,#27528);
#24911=AXIS2_PLACEMENT_3D('',#34143,#27529,#27530);
#24912=AXIS2_PLACEMENT_3D('',#34146,#27532,#27533);
#24913=AXIS2_PLACEMENT_3D('',#34147,#27534,#27535);
#24914=AXIS2_PLACEMENT_3D('',#34150,#27537,#27538);
#24915=AXIS2_PLACEMENT_3D('',#34151,#27539,#27540);
#24916=AXIS2_PLACEMENT_3D('',#34154,#27542,#27543);
#24917=AXIS2_PLACEMENT_3D('',#34155,#27544,#27545);
#24918=AXIS2_PLACEMENT_3D('',#34156,#27546,#27547);
#24919=AXIS2_PLACEMENT_3D('',#34159,#27549,#27550);
#24920=AXIS2_PLACEMENT_3D('',#34160,#27551,#27552);
#24921=AXIS2_PLACEMENT_3D('',#34163,#27554,#27555);
#24922=AXIS2_PLACEMENT_3D('',#34164,#27556,#27557);
#24923=AXIS2_PLACEMENT_3D('',#34167,#27559,#27560);
#24924=AXIS2_PLACEMENT_3D('',#34168,#27561,#27562);
#24925=AXIS2_PLACEMENT_3D('',#34169,#27563,#27564);
#24926=AXIS2_PLACEMENT_3D('',#34173,#27566,#27567);
#24927=AXIS2_PLACEMENT_3D('',#34174,#27568,#27569);
#24928=AXIS2_PLACEMENT_3D('',#34175,#27570,#27571);
#27198=DIRECTION('axis',(0.,0.,1.));
#27199=DIRECTION('refdir',(1.,0.,0.));
#27200=DIRECTION('center_axis',(0.,-5.65390683043825E-15,1.));
#27201=DIRECTION('ref_axis',(-1.,-3.05476520284318E-17,0.));
#27202=DIRECTION('center_axis',(0.,0.,1.));
#27203=DIRECTION('ref_axis',(-1.,-6.12323399573677E-17,0.));
#27204=DIRECTION('',(0.382683432365093,-5.25870392309198E-15,0.923879532511285));
#27205=DIRECTION('center_axis',(0.,0.,-1.));
#27206=DIRECTION('ref_axis',(-1.,0.,0.));
#27207=DIRECTION('center_axis',(0.,0.,-1.));
#27208=DIRECTION('ref_axis',(-1.,0.,0.));
#27209=DIRECTION('center_axis',(0.,0.,1.));
#27210=DIRECTION('ref_axis',(-1.,0.,0.));
#27211=DIRECTION('',(-0.707106781186547,-8.65956056235493E-17,-0.707106781186547));
#27212=DIRECTION('center_axis',(0.,0.,-1.));
#27213=DIRECTION('ref_axis',(-1.,-6.12323399573677E-17,0.));
#27214=DIRECTION('center_axis',(0.,0.,1.));
#27215=DIRECTION('ref_axis',(1.,0.,0.));
#27216=DIRECTION('center_axis',(0.,0.,1.));
#27217=DIRECTION('ref_axis',(1.,0.,0.));
#27218=DIRECTION('',(0.,0.,-1.));
#27219=DIRECTION('center_axis',(0.,1.35412816153563E-14,-1.));
#27220=DIRECTION('ref_axis',(-1.,-3.07842030208353E-17,0.));
#27221=DIRECTION('center_axis',(0.,0.,1.));
#27222=DIRECTION('ref_axis',(-1.,-6.12323399573677E-17,0.));
#27223=DIRECTION('',(-0.923879532511286,-5.09732241105372E-15,0.382683432365091));
#27224=DIRECTION('center_axis',(0.,0.,-1.));
#27225=DIRECTION('ref_axis',(-1.,0.,0.));
#27226=DIRECTION('center_axis',(0.,0.,-1.));
#27227=DIRECTION('ref_axis',(-1.,0.,0.));
#27228=DIRECTION('',(0.707106781186547,8.65956056235493E-17,-0.707106781186547));
#27229=DIRECTION('center_axis',(0.,0.,-1.));
#27230=DIRECTION('ref_axis',(-1.,-6.12323399573677E-17,0.));
#27231=DIRECTION('center_axis',(0.,0.,1.));
#27232=DIRECTION('ref_axis',(1.,0.,0.));
#27233=DIRECTION('center_axis',(0.,0.,1.));
#27234=DIRECTION('ref_axis',(1.,0.,0.));
#27235=DIRECTION('center_axis',(0.,0.,-1.));
#27236=DIRECTION('ref_axis',(-1.,0.,0.));
#27237=DIRECTION('center_axis',(0.,0.,-1.));
#27238=DIRECTION('ref_axis',(-1.,0.,0.));
#27239=DIRECTION('center_axis',(0.,0.,-1.));
#27240=DIRECTION('ref_axis',(-1.,0.,0.));
#27241=DIRECTION('center_axis',(0.,0.,-1.));
#27242=DIRECTION('ref_axis',(-1.,0.,0.));
#27243=DIRECTION('center_axis',(0.,0.,-1.));
#27244=DIRECTION('ref_axis',(-1.,0.,0.));
#27245=DIRECTION('center_axis',(0.,0.,-1.));
#27246=DIRECTION('ref_axis',(-1.,0.,0.));
#27247=DIRECTION('center_axis',(0.,1.35412816153564E-14,1.));
#27248=DIRECTION('ref_axis',(-1.,-3.07842030208353E-17,0.));
#27249=DIRECTION('',(-0.923879532511287,-5.32360763351127E-15,-0.38268343236509));
#27250=DIRECTION('center_axis',(0.,0.,1.));
#27251=DIRECTION('ref_axis',(-1.,0.,0.));
#27252=DIRECTION('center_axis',(0.,0.,-1.));
#27253=DIRECTION('ref_axis',(-1.,0.,0.));
#27254=DIRECTION('center_axis',(0.,0.,-1.));
#27255=DIRECTION('ref_axis',(-1.,0.,0.));
#27256=DIRECTION('center_axis',(0.,0.,-1.));
#27257=DIRECTION('ref_axis',(1.,0.,0.));
#27258=DIRECTION('center_axis',(0.,0.,-1.));
#27259=DIRECTION('ref_axis',(1.,0.,0.));
#27260=DIRECTION('center_axis',(0.,0.,-1.));
#27261=DIRECTION('ref_axis',(1.,0.,0.));
#27262=DIRECTION('center_axis',(0.,0.,-1.));
#27263=DIRECTION('ref_axis',(1.,0.,0.));
#27264=DIRECTION('center_axis',(0.,0.,-1.));
#27265=DIRECTION('ref_axis',(1.,0.,0.));
#27266=DIRECTION('center_axis',(0.,0.,-1.));
#27267=DIRECTION('ref_axis',(1.,0.,0.));
#27268=DIRECTION('center_axis',(0.,2.10365780063137E-15,-1.));
#27269=DIRECTION('ref_axis',(-1.,2.95769561248064E-17,0.));
#27270=DIRECTION('center_axis',(0.,0.,1.));
#27271=DIRECTION('ref_axis',(-1.,6.12323399573677E-17,0.));
#27272=DIRECTION('',(0.923879532511287,8.90852054498284E-16,-0.38268343236509));
#27273=DIRECTION('center_axis',(0.,0.,-1.));
#27274=DIRECTION('ref_axis',(-1.,0.,0.));
#27275=DIRECTION('',(-0.707106781186548,8.65956056235493E-17,0.707106781186548));
#27276=DIRECTION('center_axis',(0.,0.,-1.));
#27277=DIRECTION('ref_axis',(-1.,6.12323399573677E-17,0.));
#27278=DIRECTION('center_axis',(0.,-8.62308332460521E-16,-1.));
#27279=DIRECTION('ref_axis',(-1.,3.10731507051551E-17,0.));
#27280=DIRECTION('',(-0.382683432365089,8.55425403093723E-16,0.923879532511287));
#27281=DIRECTION('center_axis',(0.,0.,1.));
#27282=DIRECTION('ref_axis',(-1.,0.,0.));
#27283=DIRECTION('center_axis',(0.,0.,1.));
#27284=DIRECTION('ref_axis',(-1.,0.,0.));
#27285=DIRECTION('center_axis',(0.,0.,1.));
#27286=DIRECTION('ref_axis',(1.,0.,0.));
#27287=DIRECTION('center_axis',(0.,0.,-1.));
#27288=DIRECTION('ref_axis',(-1.,0.,0.));
#27289=DIRECTION('center_axis',(0.,0.,-1.));
#27290=DIRECTION('ref_axis',(-1.,0.,0.));
#27291=DIRECTION('',(0.,0.,-1.));
#27292=DIRECTION('center_axis',(0.,-8.62308332460519E-16,1.));
#27293=DIRECTION('ref_axis',(-1.,3.10731507051551E-17,0.));
#27294=DIRECTION('center_axis',(0.,0.,1.));
#27295=DIRECTION('ref_axis',(-1.,6.12323399573677E-17,0.));
#27296=DIRECTION('',(-0.382683432365089,7.61694994987196E-16,-0.923879532511287));
#27297=DIRECTION('center_axis',(0.,0.,1.));
#27298=DIRECTION('ref_axis',(-1.,0.,0.));
#27299=DIRECTION('',(0.707106781186548,-8.65956056235493E-17,0.707106781186548));
#27300=DIRECTION('center_axis',(0.,0.,-1.));
#27301=DIRECTION('ref_axis',(-1.,6.12323399573677E-17,0.));
#27302=DIRECTION('center_axis',(0.,2.10365780063138E-15,1.));
#27303=DIRECTION('ref_axis',(-1.,2.95769561248064E-17,0.));
#27304=DIRECTION('',(0.923879532511288,6.64566832040743E-16,0.382683432365087));
#27305=DIRECTION('center_axis',(0.,0.,1.));
#27306=DIRECTION('ref_axis',(-1.,0.,0.));
#27307=DIRECTION('center_axis',(0.,0.,1.));
#27308=DIRECTION('ref_axis',(1.,0.,0.));
#27309=DIRECTION('center_axis',(0.,0.,-1.));
#27310=DIRECTION('ref_axis',(-1.,0.,0.));
#27311=DIRECTION('center_axis',(0.,0.,-1.));
#27312=DIRECTION('ref_axis',(1.,0.,0.));
#27313=DIRECTION('center_axis',(0.,0.,-1.));
#27314=DIRECTION('ref_axis',(1.,0.,0.));
#27315=DIRECTION('center_axis',(0.,0.,-1.));
#27316=DIRECTION('ref_axis',(1.,0.,0.));
#27317=DIRECTION('center_axis',(0.,0.,-1.));
#27318=DIRECTION('ref_axis',(1.,0.,0.));
#27319=DIRECTION('',(0.70710678118655,-8.65956056235497E-17,0.707106781186545));
#27320=DIRECTION('center_axis',(0.,0.,1.));
#27321=DIRECTION('ref_axis',(1.,0.,0.));
#27322=DIRECTION('center_axis',(0.,0.,1.));
#27323=DIRECTION('ref_axis',(1.,0.,0.));
#27324=DIRECTION('center_axis',(0.,0.,-1.));
#27325=DIRECTION('ref_axis',(-1.,0.,0.));
#27326=DIRECTION('center_axis',(0.,0.,-1.));
#27327=DIRECTION('ref_axis',(1.,0.,0.));
#27328=DIRECTION('',(0.,0.,-1.));
#27329=DIRECTION('center_axis',(0.,0.,-1.));
#27330=DIRECTION('ref_axis',(1.,0.,0.));
#27331=DIRECTION('',(0.707106781186545,-8.65956056235491E-17,0.70710678118655));
#27332=DIRECTION('center_axis',(0.,0.,1.));
#27333=DIRECTION('ref_axis',(1.,0.,0.));
#27334=DIRECTION('center_axis',(0.,0.,1.));
#27335=DIRECTION('ref_axis',(1.,0.,0.));
#27336=DIRECTION('center_axis',(0.,0.,-1.));
#27337=DIRECTION('ref_axis',(-1.,0.,0.));
#27338=DIRECTION('center_axis',(0.,0.,-1.));
#27339=DIRECTION('ref_axis',(1.,0.,0.));
#27340=DIRECTION('',(0.,0.,-1.));
#27341=DIRECTION('center_axis',(0.,0.,-1.));
#27342=DIRECTION('ref_axis',(1.,0.,0.));
#27343=DIRECTION('',(0.707106781186548,-8.65956056235494E-17,0.707106781186547));
#27344=DIRECTION('center_axis',(0.,0.,1.));
#27345=DIRECTION('ref_axis',(1.,0.,0.));
#27346=DIRECTION('center_axis',(0.,0.,1.));
#27347=DIRECTION('ref_axis',(1.,0.,0.));
#27348=DIRECTION('center_axis',(0.,0.,-1.));
#27349=DIRECTION('ref_axis',(-1.,0.,0.));
#27350=DIRECTION('center_axis',(0.,0.,-1.));
#27351=DIRECTION('ref_axis',(1.,0.,0.));
#27352=DIRECTION('',(0.,0.,-1.));
#27353=DIRECTION('center_axis',(0.,0.,-1.));
#27354=DIRECTION('ref_axis',(1.,0.,0.));
#27355=DIRECTION('',(0.70710678118655,-8.65956056235497E-17,0.707106781186545));
#27356=DIRECTION('center_axis',(0.,0.,1.));
#27357=DIRECTION('ref_axis',(1.,0.,0.));
#27358=DIRECTION('center_axis',(0.,0.,1.));
#27359=DIRECTION('ref_axis',(1.,0.,0.));
#27360=DIRECTION('center_axis',(0.,0.,-1.));
#27361=DIRECTION('ref_axis',(-1.,0.,0.));
#27362=DIRECTION('center_axis',(0.,0.,-1.));
#27363=DIRECTION('ref_axis',(1.,0.,0.));
#27364=DIRECTION('',(0.,0.,-1.));
#27365=DIRECTION('center_axis',(0.,0.,-1.));
#27366=DIRECTION('ref_axis',(1.,0.,0.));
#27367=DIRECTION('',(0.707106781186548,-8.65956056235494E-17,0.707106781186547));
#27368=DIRECTION('center_axis',(0.,0.,1.));
#27369=DIRECTION('ref_axis',(1.,0.,0.));
#27370=DIRECTION('center_axis',(0.,0.,1.));
#27371=DIRECTION('ref_axis',(1.,0.,0.));
#27372=DIRECTION('center_axis',(0.,0.,-1.));
#27373=DIRECTION('ref_axis',(-1.,0.,0.));
#27374=DIRECTION('center_axis',(0.,0.,-1.));
#27375=DIRECTION('ref_axis',(1.,0.,0.));
#27376=DIRECTION('',(0.,0.,-1.));
#27377=DIRECTION('center_axis',(0.,0.,-1.));
#27378=DIRECTION('ref_axis',(1.,0.,0.));
#27379=DIRECTION('',(0.707106781186545,-8.65956056235491E-17,0.70710678118655));
#27380=DIRECTION('center_axis',(0.,0.,1.));
#27381=DIRECTION('ref_axis',(1.,0.,0.));
#27382=DIRECTION('center_axis',(0.,0.,1.));
#27383=DIRECTION('ref_axis',(1.,0.,0.));
#27384=DIRECTION('center_axis',(0.,0.,-1.));
#27385=DIRECTION('ref_axis',(-1.,0.,0.));
#27386=DIRECTION('center_axis',(0.,0.,-1.));
#27387=DIRECTION('ref_axis',(1.,0.,0.));
#27388=DIRECTION('',(0.,0.,-1.));
#27389=DIRECTION('center_axis',(0.,-5.65390683043823E-15,-1.));
#27390=DIRECTION('ref_axis',(-1.,-3.05476520284318E-17,0.));
#27391=DIRECTION('',(0.382683432365092,-5.16497351498544E-15,-0.923879532511286));
#27392=DIRECTION('center_axis',(0.,0.,1.));
#27393=DIRECTION('ref_axis',(-1.,0.,0.));
#27394=DIRECTION('center_axis',(0.,0.,1.));
#27395=DIRECTION('ref_axis',(-1.,0.,0.));
#27396=DIRECTION('center_axis',(0.,0.,1.));
#27397=DIRECTION('ref_axis',(1.,0.,0.));
#27398=DIRECTION('',(0.,0.,-1.));
#27399=DIRECTION('center_axis',(0.,0.,-1.));
#27400=DIRECTION('ref_axis',(1.,0.,0.));
#27401=DIRECTION('center_axis',(0.,0.,1.));
#27402=DIRECTION('ref_axis',(1.,0.,0.));
#27403=DIRECTION('',(0.70710678118655,8.65956056235496E-17,-0.707106781186545));
#27404=DIRECTION('center_axis',(0.,0.,1.));
#27405=DIRECTION('ref_axis',(1.,0.,0.));
#27406=DIRECTION('center_axis',(0.,0.,1.));
#27407=DIRECTION('ref_axis',(1.,0.,0.));
#27408=DIRECTION('center_axis',(0.,0.,1.));
#27409=DIRECTION('ref_axis',(1.,0.,0.));
#27410=DIRECTION('center_axis',(0.,0.,-1.));
#27411=DIRECTION('ref_axis',(1.,0.,0.));
#27412=DIRECTION('',(0.70710678118655,-8.65956056235496E-17,0.707106781186545));
#27413=DIRECTION('center_axis',(0.,0.,-1.));
#27414=DIRECTION('ref_axis',(1.,0.,0.));
#27415=DIRECTION('center_axis',(0.,0.,-1.));
#27416=DIRECTION('ref_axis',(-1.,0.,0.));
#27417=DIRECTION('center_axis',(0.,0.,1.));
#27418=DIRECTION('ref_axis',(1.,0.,0.));
#27419=DIRECTION('center_axis',(0.,0.,1.));
#27420=DIRECTION('ref_axis',(1.,0.,0.));
#27421=DIRECTION('',(0.,0.,1.));
#27422=DIRECTION('center_axis',(0.,0.,1.));
#27423=DIRECTION('ref_axis',(1.,0.,0.));
#27424=DIRECTION('',(-0.857167300702112,-1.04972719113862E-16,0.515038074910054));
#27425=DIRECTION('center_axis',(0.,0.,1.));
#27426=DIRECTION('ref_axis',(1.,0.,0.));
#27427=DIRECTION('center_axis',(0.,0.,1.));
#27428=DIRECTION('ref_axis',(1.,0.,0.));
#27429=DIRECTION('',(0.,0.,1.));
#27430=DIRECTION('center_axis',(0.,0.,1.));
#27431=DIRECTION('ref_axis',(1.,0.,0.));
#27432=DIRECTION('center_axis',(0.,0.,1.));
#27433=DIRECTION('ref_axis',(1.,0.,0.));
#27434=DIRECTION('',(-0.707106781186548,-8.65956056235494E-17,0.707106781186547));
#27435=DIRECTION('center_axis',(0.,0.,1.));
#27436=DIRECTION('ref_axis',(1.,0.,0.));
#27437=DIRECTION('',(-0.857167300702112,-1.04972719113862E-16,0.515038074910054));
#27438=DIRECTION('center_axis',(0.,0.,1.));
#27439=DIRECTION('ref_axis',(1.,0.,0.));
#27440=DIRECTION('center_axis',(0.,0.,1.));
#27441=DIRECTION('ref_axis',(1.,0.,0.));
#27442=DIRECTION('',(0.,0.,1.));
#27443=DIRECTION('center_axis',(0.,0.,1.));
#27444=DIRECTION('ref_axis',(1.,0.,0.));
#27445=DIRECTION('center_axis',(0.,0.,1.));
#27446=DIRECTION('ref_axis',(1.,0.,0.));
#27447=DIRECTION('',(-0.707106781186548,-8.65956056235494E-17,0.707106781186547));
#27448=DIRECTION('center_axis',(0.,0.,1.));
#27449=DIRECTION('ref_axis',(1.,0.,0.));
#27450=DIRECTION('',(-0.857167300702113,-1.04972719113862E-16,0.515038074910054));
#27451=DIRECTION('center_axis',(0.,0.,1.));
#27452=DIRECTION('ref_axis',(1.,0.,0.));
#27453=DIRECTION('center_axis',(0.,0.,1.));
#27454=DIRECTION('ref_axis',(1.,0.,0.));
#27455=DIRECTION('',(0.,0.,1.));
#27456=DIRECTION('center_axis',(0.,0.,1.));
#27457=DIRECTION('ref_axis',(1.,0.,0.));
#27458=DIRECTION('center_axis',(0.,0.,1.));
#27459=DIRECTION('ref_axis',(1.,0.,0.));
#27460=DIRECTION('',(-0.707106781186548,-8.65956056235494E-17,0.707106781186547));
#27461=DIRECTION('center_axis',(0.,0.,1.));
#27462=DIRECTION('ref_axis',(-1.,0.,0.));
#27463=DIRECTION('',(-0.316227766016837,3.87267321454038E-17,-0.948683298050514));
#27464=DIRECTION('center_axis',(0.,0.,-1.));
#27465=DIRECTION('ref_axis',(1.,0.,0.));
#27466=DIRECTION('center_axis',(0.,0.,-1.));
#27467=DIRECTION('ref_axis',(-1.,0.,0.));
#27468=DIRECTION('',(0.,0.,-1.));
#27469=DIRECTION('center_axis',(0.,0.,-1.));
#27470=DIRECTION('ref_axis',(1.,0.,0.));
#27471=DIRECTION('center_axis',(0.,0.,-1.));
#27472=DIRECTION('ref_axis',(-1.,0.,0.));
#27473=DIRECTION('',(0.707106781186546,-8.65956056235491E-17,-0.707106781186549));
#27474=DIRECTION('center_axis',(0.,0.,-1.));
#27475=DIRECTION('ref_axis',(1.,0.,0.));
#27476=DIRECTION('center_axis',(0.,0.,1.));
#27477=DIRECTION('ref_axis',(1.,0.,0.));
#27478=DIRECTION('center_axis',(0.,0.,1.));
#27479=DIRECTION('ref_axis',(-1.,0.,0.));
#27480=DIRECTION('',(-0.316227766016837,3.87267321454038E-17,-0.948683298050514));
#27481=DIRECTION('center_axis',(0.,0.,-1.));
#27482=DIRECTION('ref_axis',(1.,0.,0.));
#27483=DIRECTION('center_axis',(0.,0.,-1.));
#27484=DIRECTION('ref_axis',(-1.,0.,0.));
#27485=DIRECTION('',(0.,0.,-1.));
#27486=DIRECTION('center_axis',(0.,0.,-1.));
#27487=DIRECTION('ref_axis',(1.,0.,0.));
#27488=DIRECTION('center_axis',(0.,0.,-1.));
#27489=DIRECTION('ref_axis',(-1.,0.,0.));
#27490=DIRECTION('',(0.707106781186546,-8.65956056235492E-17,-0.707106781186549));
#27491=DIRECTION('center_axis',(0.,0.,-1.));
#27492=DIRECTION('ref_axis',(1.,0.,0.));
#27493=DIRECTION('center_axis',(0.,0.,1.));
#27494=DIRECTION('ref_axis',(1.,0.,0.));
#27495=DIRECTION('center_axis',(0.,0.,1.));
#27496=DIRECTION('ref_axis',(-1.,0.,0.));
#27497=DIRECTION('',(-0.316227766016842,3.87267321454044E-17,-0.948683298050512));
#27498=DIRECTION('center_axis',(0.,0.,-1.));
#27499=DIRECTION('ref_axis',(1.,0.,0.));
#27500=DIRECTION('center_axis',(0.,0.,-1.));
#27501=DIRECTION('ref_axis',(-1.,0.,0.));
#27502=DIRECTION('',(0.,0.,-1.));
#27503=DIRECTION('center_axis',(0.,0.,-1.));
#27504=DIRECTION('ref_axis',(1.,0.,0.));
#27505=DIRECTION('center_axis',(0.,0.,-1.));
#27506=DIRECTION('ref_axis',(-1.,0.,0.));
#27507=DIRECTION('',(0.707106781186552,-8.65956056235499E-17,-0.707106781186543));
#27508=DIRECTION('center_axis',(0.,0.,-1.));
#27509=DIRECTION('ref_axis',(1.,0.,0.));
#27510=DIRECTION('center_axis',(0.,0.,1.));
#27511=DIRECTION('ref_axis',(1.,0.,0.));
#27512=DIRECTION('center_axis',(0.,0.,1.));
#27513=DIRECTION('ref_axis',(-1.,0.,0.));
#27514=DIRECTION('',(-0.316227766016837,3.87267321454038E-17,-0.948683298050514));
#27515=DIRECTION('center_axis',(0.,0.,-1.));
#27516=DIRECTION('ref_axis',(1.,0.,0.));
#27517=DIRECTION('center_axis',(0.,0.,-1.));
#27518=DIRECTION('ref_axis',(-1.,0.,0.));
#27519=DIRECTION('',(0.,0.,-1.));
#27520=DIRECTION('center_axis',(0.,0.,-1.));
#27521=DIRECTION('ref_axis',(1.,0.,0.));
#27522=DIRECTION('center_axis',(0.,0.,-1.));
#27523=DIRECTION('ref_axis',(-1.,0.,0.));
#27524=DIRECTION('',(0.707106781186546,-8.65956056235492E-17,-0.707106781186549));
#27525=DIRECTION('center_axis',(0.,0.,-1.));
#27526=DIRECTION('ref_axis',(1.,0.,0.));
#27527=DIRECTION('center_axis',(0.,0.,1.));
#27528=DIRECTION('ref_axis',(1.,0.,0.));
#27529=DIRECTION('center_axis',(0.,0.,1.));
#27530=DIRECTION('ref_axis',(-1.,0.,0.));
#27531=DIRECTION('',(-0.316227766016837,3.87267321454038E-17,-0.948683298050514));
#27532=DIRECTION('center_axis',(0.,0.,-1.));
#27533=DIRECTION('ref_axis',(1.,0.,0.));
#27534=DIRECTION('center_axis',(0.,0.,-1.));
#27535=DIRECTION('ref_axis',(-1.,0.,0.));
#27536=DIRECTION('',(0.,0.,-1.));
#27537=DIRECTION('center_axis',(0.,0.,-1.));
#27538=DIRECTION('ref_axis',(1.,0.,0.));
#27539=DIRECTION('center_axis',(0.,0.,-1.));
#27540=DIRECTION('ref_axis',(-1.,0.,0.));
#27541=DIRECTION('',(0.707106781186546,-8.65956056235491E-17,-0.707106781186549));
#27542=DIRECTION('center_axis',(0.,0.,-1.));
#27543=DIRECTION('ref_axis',(1.,0.,0.));
#27544=DIRECTION('center_axis',(0.,0.,1.));
#27545=DIRECTION('ref_axis',(1.,0.,0.));
#27546=DIRECTION('center_axis',(0.,0.,1.));
#27547=DIRECTION('ref_axis',(-1.,0.,0.));
#27548=DIRECTION('',(-0.316227766016842,3.87267321454044E-17,-0.948683298050512));
#27549=DIRECTION('center_axis',(0.,0.,-1.));
#27550=DIRECTION('ref_axis',(1.,0.,0.));
#27551=DIRECTION('center_axis',(0.,0.,-1.));
#27552=DIRECTION('ref_axis',(-1.,0.,0.));
#27553=DIRECTION('',(0.,0.,-1.));
#27554=DIRECTION('center_axis',(0.,0.,-1.));
#27555=DIRECTION('ref_axis',(1.,0.,0.));
#27556=DIRECTION('center_axis',(0.,0.,-1.));
#27557=DIRECTION('ref_axis',(-1.,0.,0.));
#27558=DIRECTION('',(0.707106781186552,-8.65956056235499E-17,-0.707106781186543));
#27559=DIRECTION('center_axis',(0.,0.,-1.));
#27560=DIRECTION('ref_axis',(1.,0.,0.));
#27561=DIRECTION('center_axis',(0.,0.,1.));
#27562=DIRECTION('ref_axis',(1.,0.,0.));
#27563=DIRECTION('center_axis',(0.,0.,-1.));
#27564=DIRECTION('ref_axis',(-1.,0.,0.));
#27565=DIRECTION('',(0.707106781186548,8.65956056235493E-17,-0.707106781186548));
#27566=DIRECTION('center_axis',(0.,0.,1.));
#27567=DIRECTION('ref_axis',(-1.,0.,0.));
#27568=DIRECTION('center_axis',(0.,0.,1.));
#27569=DIRECTION('ref_axis',(-1.,0.,0.));
#27570=DIRECTION('center_axis',(0.,0.,1.));
#27571=DIRECTION('ref_axis',(1.,0.,0.));
#27572=DIRECTION('',(0.,0.,-1.));
#33870=CARTESIAN_POINT('',(0.,0.,0.));
#33871=CARTESIAN_POINT('Origin',(0.,1.44777340356572E-16,0.0843933982822012));
#33872=CARTESIAN_POINT('',(4.7287867965644,1.15821872285257E-15,0.0587867965644029));
#33873=CARTESIAN_POINT('Origin',(0.,2.89554680713143E-16,0.0587867965644029));
#33874=CARTESIAN_POINT('',(4.75,-5.81707229594993E-16,0.11));
#33875=CARTESIAN_POINT('',(4.7393933982822,-2.90853614797496E-16,0.0843933982822012));
#33876=CARTESIAN_POINT('',(-4.75,-5.81707229594993E-16,0.11));
#33877=CARTESIAN_POINT('Origin',(0.,0.,0.11));
#33878=CARTESIAN_POINT('Origin',(0.,0.,0.11));
#33879=CARTESIAN_POINT('Origin',(0.,0.,0.04));
#33880=CARTESIAN_POINT('',(4.6912132034356,0.,0.0212132034355967));
#33881=CARTESIAN_POINT('',(4.71,5.76808642398403E-16,0.04));
#33882=CARTESIAN_POINT('Origin',(0.,2.8725396168526E-16,0.0212132034355967));
#33883=CARTESIAN_POINT('Origin',(0.,0.,0.7));
#33884=CARTESIAN_POINT('',(-4.75,-5.81707229594993E-16,0.65));
#33885=CARTESIAN_POINT('Origin',(0.,0.,0.65));
#33886=CARTESIAN_POINT('',(-4.75,-5.81707229594993E-16,0.7));
#33887=CARTESIAN_POINT('Origin',(0.,1.4362698084263E-16,1.3893933982822));
#33888=CARTESIAN_POINT('',(4.6912132034356,1.14901584674104E-15,1.3787867965644));
#33889=CARTESIAN_POINT('Origin',(0.,2.8725396168526E-16,1.3787867965644));
#33890=CARTESIAN_POINT('',(4.64,-5.68236114804372E-16,1.4));
#33891=CARTESIAN_POINT('',(4.6656066017178,-2.84118057402186E-16,1.3893933982822));
#33892=CARTESIAN_POINT('Origin',(0.,0.,1.4));
#33893=CARTESIAN_POINT('Origin',(0.,0.,1.36));
#33894=CARTESIAN_POINT('',(4.7287867965644,0.,1.3412132034356));
#33895=CARTESIAN_POINT('',(4.71,5.76808642398403E-16,1.36));
#33896=CARTESIAN_POINT('Origin',(0.,2.89554680713143E-16,1.3412132034356));
#33897=CARTESIAN_POINT('Origin',(4.095,0.,1.4));
#33898=CARTESIAN_POINT('',(-4.095,-5.01492864250841E-16,1.4));
#33899=CARTESIAN_POINT('Origin',(0.,0.,1.4));
#33900=CARTESIAN_POINT('',(4.44833333333333,-1.57163005890577E-17,1.4));
#33901=CARTESIAN_POINT('Origin',(4.32,0.,1.4));
#33902=CARTESIAN_POINT('',(2.28833333333333,3.74122974434878,1.4));
#33903=CARTESIAN_POINT('Origin',(2.16,3.74122974434878,1.4));
#33904=CARTESIAN_POINT('',(-2.03166666666667,3.74122974434878,1.4));
#33905=CARTESIAN_POINT('Origin',(-2.16,3.74122974434878,1.4));
#33906=CARTESIAN_POINT('',(-4.19166666666667,5.13331116642599E-16,1.4));
#33907=CARTESIAN_POINT('Origin',(-4.32,5.29047417231657E-16,1.4));
#33908=CARTESIAN_POINT('',(-2.03166666666667,-3.74122974434877,1.4));
#33909=CARTESIAN_POINT('Origin',(-2.16,-3.74122974434877,1.4));
#33910=CARTESIAN_POINT('',(2.28833333333333,-3.74122974434878,1.4));
#33911=CARTESIAN_POINT('Origin',(2.16,-3.74122974434878,1.4));
#33912=CARTESIAN_POINT('Origin',(0.,1.4362698084263E-16,0.0106066017177983));
#33913=CARTESIAN_POINT('',(4.64,5.68236114804372E-16,0.));
#33914=CARTESIAN_POINT('',(4.6656066017178,8.58625980772706E-16,0.0106066017177983));
#33915=CARTESIAN_POINT('Origin',(0.,0.,0.));
#33916=CARTESIAN_POINT('Origin',(4.75,0.,0.));
#33917=CARTESIAN_POINT('',(0.78,-9.55224503334935E-17,0.));
#33918=CARTESIAN_POINT('Origin',(0.,0.,0.));
#33919=CARTESIAN_POINT('',(1.92,3.74122974434878,0.));
#33920=CARTESIAN_POINT('Origin',(2.16,3.74122974434878,0.));
#33921=CARTESIAN_POINT('',(-4.56,5.58438940411193E-16,0.));
#33922=CARTESIAN_POINT('Origin',(-4.32,5.29047417231657E-16,0.));
#33923=CARTESIAN_POINT('',(1.92,-3.74122974434878,0.));
#33924=CARTESIAN_POINT('Origin',(2.16,-3.74122974434878,0.));
#33925=CARTESIAN_POINT('',(-2.4,-3.74122974434877,0.));
#33926=CARTESIAN_POINT('Origin',(-2.16,-3.74122974434877,0.));
#33927=CARTESIAN_POINT('',(-2.4,3.74122974434878,0.));
#33928=CARTESIAN_POINT('Origin',(-2.16,3.74122974434878,0.));
#33929=CARTESIAN_POINT('',(4.08,2.93915231795365E-17,0.));
#33930=CARTESIAN_POINT('Origin',(4.32,0.,0.));
#33931=CARTESIAN_POINT('Origin',(0.,-2.23126604418363E-17,0.0106066017177982));
#33932=CARTESIAN_POINT('',(0.728786796564404,0.,0.0212132034355964));
#33933=CARTESIAN_POINT('Origin',(0.,-4.46253208836725E-17,0.0212132034355964));
#33934=CARTESIAN_POINT('',(0.754393398282202,4.77612251667468E-17,0.0106066017177982));
#33935=CARTESIAN_POINT('Origin',(0.,0.,0.025));
#33936=CARTESIAN_POINT('',(0.721213203435596,-1.76646288218042E-16,0.0287867965644036));
#33937=CARTESIAN_POINT('',(0.725,-8.87868929381831E-17,0.025));
#33938=CARTESIAN_POINT('Origin',(0.,-4.41615720545106E-17,0.0287867965644036));
#33939=CARTESIAN_POINT('Origin',(0.,-2.20807860272553E-17,0.0543933982822019));
#33940=CARTESIAN_POINT('',(0.7,8.57252759403147E-17,0.0800000000000001));
#33941=CARTESIAN_POINT('',(0.710606601717798,-1.31185782079179E-16,0.0543933982822019));
#33942=CARTESIAN_POINT('',(-0.7,-8.57252759403147E-17,0.0800000000000001));
#33943=CARTESIAN_POINT('Origin',(0.,0.,0.0800000000000001));
#33944=CARTESIAN_POINT('Origin',(0.,0.,0.0800000000000001));
#33945=CARTESIAN_POINT('Origin',(0.,0.,1.));
#33946=CARTESIAN_POINT('',(0.7,-8.57252759403147E-17,1.92));
#33947=CARTESIAN_POINT('',(-0.7,-8.57252759403147E-17,1.92));
#33948=CARTESIAN_POINT('Origin',(0.,0.,1.92));
#33949=CARTESIAN_POINT('Origin',(0.,0.,1.92));
#33950=CARTESIAN_POINT('',(-0.7,-8.57252759403147E-17,1.));
#33951=CARTESIAN_POINT('Origin',(0.,-2.20807860272553E-17,1.9456066017178));
#33952=CARTESIAN_POINT('',(0.721213203435596,0.,1.9712132034356));
#33953=CARTESIAN_POINT('Origin',(0.,-4.41615720545106E-17,1.9712132034356));
#33954=CARTESIAN_POINT('',(0.710606601717798,4.28626379701574E-17,1.9456066017178));
#33955=CARTESIAN_POINT('Origin',(0.,0.,1.975));
#33956=CARTESIAN_POINT('',(0.728786796564404,-1.7850128353469E-16,1.9787867965644));
#33957=CARTESIAN_POINT('',(0.725,-8.87868929381831E-17,1.975));
#33958=CARTESIAN_POINT('Origin',(0.,-4.46253208836725E-17,1.9787867965644));
#33959=CARTESIAN_POINT('Origin',(0.,-2.23126604418363E-17,1.9893933982822));
#33960=CARTESIAN_POINT('',(0.78,9.55224503334936E-17,2.));
#33961=CARTESIAN_POINT('',(0.754393398282202,-1.37011866934092E-16,1.9893933982822));
#33962=CARTESIAN_POINT('Origin',(0.,0.,2.));
#33963=CARTESIAN_POINT('Origin',(0.7,0.,2.));
#33964=CARTESIAN_POINT('',(4.055,-4.96594277054252E-16,2.));
#33965=CARTESIAN_POINT('Origin',(0.,0.,2.));
#33966=CARTESIAN_POINT('',(-0.18,3.4,2.));
#33967=CARTESIAN_POINT('Origin',(2.0818995585505E-16,3.4,2.));
#33968=CARTESIAN_POINT('',(-3.12448637286709,-1.7,2.));
#33969=CARTESIAN_POINT('Origin',(-2.94448637286709,-1.7,2.));
#33970=CARTESIAN_POINT('',(2.76448637286709,-1.7,2.));
#33971=CARTESIAN_POINT('Origin',(2.94448637286709,-1.7,2.));
#33972=CARTESIAN_POINT('Origin',(4.32,0.,0.015));
#33973=CARTESIAN_POINT('',(4.11,-2.57175827820944E-17,0.03));
#33974=CARTESIAN_POINT('',(4.095,2.75545529808155E-17,0.015));
#33975=CARTESIAN_POINT('',(4.53,-2.57175827820944E-17,0.03));
#33976=CARTESIAN_POINT('Origin',(4.32,0.,0.03));
#33977=CARTESIAN_POINT('Origin',(4.32,0.,0.03));
#33978=CARTESIAN_POINT('Origin',(4.32,0.,0.25));
#33979=CARTESIAN_POINT('',(4.53,-2.57175827820944E-17,0.5));
#33980=CARTESIAN_POINT('Origin',(4.32,0.,0.5));
#33981=CARTESIAN_POINT('',(4.53,-2.57175827820944E-17,0.25));
#33982=CARTESIAN_POINT('Origin',(2.16,3.74122974434878,0.015));
#33983=CARTESIAN_POINT('',(1.95,3.74122974434878,0.03));
#33984=CARTESIAN_POINT('',(1.935,3.74122974434878,0.015));
#33985=CARTESIAN_POINT('',(2.37,3.74122974434878,0.03));
#33986=CARTESIAN_POINT('Origin',(2.16,3.74122974434878,0.03));
#33987=CARTESIAN_POINT('Origin',(2.16,3.74122974434878,0.03));
#33988=CARTESIAN_POINT('Origin',(2.16,3.74122974434878,0.25));
#33989=CARTESIAN_POINT('',(2.37,3.74122974434878,0.5));
#33990=CARTESIAN_POINT('Origin',(2.16,3.74122974434878,0.5));
#33991=CARTESIAN_POINT('',(2.37,3.74122974434878,0.25));
#33992=CARTESIAN_POINT('Origin',(-2.16,3.74122974434878,0.015));
#33993=CARTESIAN_POINT('',(-2.37,3.74122974434878,0.03));
#33994=CARTESIAN_POINT('',(-2.385,3.74122974434878,0.015));
#33995=CARTESIAN_POINT('',(-1.95,3.74122974434878,0.03));
#33996=CARTESIAN_POINT('Origin',(-2.16,3.74122974434878,0.03));
#33997=CARTESIAN_POINT('Origin',(-2.16,3.74122974434878,0.03));
#33998=CARTESIAN_POINT('Origin',(-2.16,3.74122974434878,0.25));
#33999=CARTESIAN_POINT('',(-1.95,3.74122974434878,0.5));
#34000=CARTESIAN_POINT('Origin',(-2.16,3.74122974434878,0.5));
#34001=CARTESIAN_POINT('',(-1.95,3.74122974434878,0.25));
#34002=CARTESIAN_POINT('Origin',(-4.32,5.29047417231657E-16,0.015));
#34003=CARTESIAN_POINT('',(-4.53,5.03329834449562E-16,0.03));
#34004=CARTESIAN_POINT('',(-4.545,5.56601970212472E-16,0.015));
#34005=CARTESIAN_POINT('',(-4.11,5.03329834449562E-16,0.03));
#34006=CARTESIAN_POINT('Origin',(-4.32,5.29047417231657E-16,0.03));
#34007=CARTESIAN_POINT('Origin',(-4.32,5.29047417231657E-16,0.03));
#34008=CARTESIAN_POINT('Origin',(-4.32,5.29047417231657E-16,0.25));
#34009=CARTESIAN_POINT('',(-4.11,5.03329834449562E-16,0.5));
#34010=CARTESIAN_POINT('Origin',(-4.32,5.29047417231657E-16,0.5));
#34011=CARTESIAN_POINT('',(-4.11,5.03329834449562E-16,0.25));
#34012=CARTESIAN_POINT('Origin',(-2.16,-3.74122974434877,0.015));
#34013=CARTESIAN_POINT('',(-2.37,-3.74122974434877,0.03));
#34014=CARTESIAN_POINT('',(-2.385,-3.74122974434877,0.015));
#34015=CARTESIAN_POINT('',(-1.95,-3.74122974434877,0.03));
#34016=CARTESIAN_POINT('Origin',(-2.16,-3.74122974434877,0.03));
#34017=CARTESIAN_POINT('Origin',(-2.16,-3.74122974434877,0.03));
#34018=CARTESIAN_POINT('Origin',(-2.16,-3.74122974434877,0.25));
#34019=CARTESIAN_POINT('',(-1.95,-3.74122974434877,0.5));
#34020=CARTESIAN_POINT('Origin',(-2.16,-3.74122974434877,0.5));
#34021=CARTESIAN_POINT('',(-1.95,-3.74122974434877,0.25));
#34022=CARTESIAN_POINT('Origin',(2.16,-3.74122974434878,0.015));
#34023=CARTESIAN_POINT('',(1.95,-3.74122974434878,0.03));
#34024=CARTESIAN_POINT('',(1.935,-3.74122974434878,0.015));
#34025=CARTESIAN_POINT('',(2.37,-3.74122974434878,0.03));
#34026=CARTESIAN_POINT('Origin',(2.16,-3.74122974434878,0.03));
#34027=CARTESIAN_POINT('Origin',(2.16,-3.74122974434878,0.03));
#34028=CARTESIAN_POINT('Origin',(2.16,-3.74122974434878,0.25));
#34029=CARTESIAN_POINT('',(2.37,-3.74122974434878,0.5));
#34030=CARTESIAN_POINT('Origin',(2.16,-3.74122974434878,0.5));
#34031=CARTESIAN_POINT('',(2.37,-3.74122974434878,0.25));
#34032=CARTESIAN_POINT('Origin',(0.,1.44777340356572E-16,1.3156066017178));
#34033=CARTESIAN_POINT('',(4.75,5.81707229594993E-16,1.29));
#34034=CARTESIAN_POINT('',(4.7393933982822,8.69962976223783E-16,1.3156066017178));
#34035=CARTESIAN_POINT('',(-4.75,-5.81707229594993E-16,1.29));
#34036=CARTESIAN_POINT('Origin',(0.,0.,1.29));
#34037=CARTESIAN_POINT('Origin',(0.,0.,1.29));
#34038=CARTESIAN_POINT('Origin',(0.,0.,0.7));
#34039=CARTESIAN_POINT('',(-4.75,5.81707229594993E-16,0.77));
#34040=CARTESIAN_POINT('',(-4.75,-5.81707229594993E-16,0.7));
#34041=CARTESIAN_POINT('Origin',(0.,0.,0.77));
#34042=CARTESIAN_POINT('Origin',(0.,0.,0.755));
#34043=CARTESIAN_POINT('',(-4.72,-5.78033289197551E-16,0.74));
#34044=CARTESIAN_POINT('',(-4.735,-5.79870259396272E-16,0.755));
#34045=CARTESIAN_POINT('Origin',(0.,0.,0.74));
#34046=CARTESIAN_POINT('Origin',(4.66,0.,0.74));
#34047=CARTESIAN_POINT('',(-4.66,-5.70685408402667E-16,0.74));
#34048=CARTESIAN_POINT('Origin',(0.,0.,0.74));
#34049=CARTESIAN_POINT('Origin',(0.,0.,0.665));
#34050=CARTESIAN_POINT('',(-4.72,5.78033289197551E-16,0.68));
#34051=CARTESIAN_POINT('',(-4.735,5.79870259396272E-16,0.665));
#34052=CARTESIAN_POINT('Origin',(0.,0.,0.68));
#34053=CARTESIAN_POINT('Origin',(4.8,0.,0.68));
#34054=CARTESIAN_POINT('',(-4.66,-5.70685408402667E-16,0.68));
#34055=CARTESIAN_POINT('Origin',(0.,0.,0.68));
#34056=CARTESIAN_POINT('Origin',(0.,0.,0.71));
#34057=CARTESIAN_POINT('',(-4.66,-5.70685408402667E-16,0.71));
#34058=CARTESIAN_POINT('Origin',(2.94448637286709,-1.7,1.36094405976321));
#34059=CARTESIAN_POINT('',(2.94448637286709,-1.7,1.32188811952642));
#34060=CARTESIAN_POINT('',(2.81448637286709,-1.7,1.4));
#34061=CARTESIAN_POINT('',(2.87948637286709,-1.7,1.36094405976321));
#34062=CARTESIAN_POINT('Origin',(2.94448637286709,-1.7,1.4));
#34063=CARTESIAN_POINT('Origin',(2.94448637286709,-1.7,1.675));
#34064=CARTESIAN_POINT('',(2.81448637286709,-1.7,1.95));
#34065=CARTESIAN_POINT('',(2.81448637286709,-1.7,1.675));
#34066=CARTESIAN_POINT('Origin',(2.94448637286709,-1.7,1.95));
#34067=CARTESIAN_POINT('Origin',(2.94448637286709,-1.7,2.));
#34068=CARTESIAN_POINT('',(2.76448637286709,-1.7,2.));
#34069=CARTESIAN_POINT('Origin',(-2.94448637286709,-1.7,1.36094405976321));
#34070=CARTESIAN_POINT('',(-2.94448637286709,-1.7,1.32188811952642));
#34071=CARTESIAN_POINT('',(-3.07448637286709,-1.7,1.4));
#34072=CARTESIAN_POINT('',(-3.00948637286709,-1.7,1.36094405976321));
#34073=CARTESIAN_POINT('Origin',(-2.94448637286709,-1.7,1.4));
#34074=CARTESIAN_POINT('Origin',(-2.94448637286709,-1.7,1.675));
#34075=CARTESIAN_POINT('',(-3.07448637286709,-1.7,1.95));
#34076=CARTESIAN_POINT('',(-3.07448637286709,-1.7,1.675));
#34077=CARTESIAN_POINT('Origin',(-2.94448637286709,-1.7,1.95));
#34078=CARTESIAN_POINT('Origin',(-2.94448637286709,-1.7,2.));
#34079=CARTESIAN_POINT('',(-3.12448637286709,-1.7,2.));
#34080=CARTESIAN_POINT('Origin',(2.0818995585505E-16,3.4,1.36094405976321));
#34081=CARTESIAN_POINT('',(2.0818995585505E-16,3.4,1.32188811952642));
#34082=CARTESIAN_POINT('',(-0.13,3.4,1.4));
#34083=CARTESIAN_POINT('',(-0.0649999999999998,3.4,1.36094405976321));
#34084=CARTESIAN_POINT('Origin',(2.0818995585505E-16,3.4,1.4));
#34085=CARTESIAN_POINT('Origin',(2.0818995585505E-16,3.4,1.675));
#34086=CARTESIAN_POINT('',(-0.13,3.4,1.95));
#34087=CARTESIAN_POINT('',(-0.13,3.4,1.675));
#34088=CARTESIAN_POINT('Origin',(2.0818995585505E-16,3.4,1.95));
#34089=CARTESIAN_POINT('Origin',(2.0818995585505E-16,3.4,2.));
#34090=CARTESIAN_POINT('',(-0.18,3.4,2.));
#34091=CARTESIAN_POINT('Origin',(2.16,-3.74122974434878,1.4125));
#34092=CARTESIAN_POINT('',(2.28,-3.74122974434878,1.375));
#34093=CARTESIAN_POINT('',(2.2925,-3.74122974434878,1.4125));
#34094=CARTESIAN_POINT('Origin',(2.16,-3.74122974434878,1.375));
#34095=CARTESIAN_POINT('Origin',(2.16,-3.74122974434878,0.95));
#34096=CARTESIAN_POINT('',(2.28,-3.74122974434878,0.525));
#34097=CARTESIAN_POINT('',(2.28,-3.74122974434878,0.95));
#34098=CARTESIAN_POINT('Origin',(2.16,-3.74122974434878,0.525));
#34099=CARTESIAN_POINT('Origin',(2.16,-3.74122974434878,0.5125));
#34100=CARTESIAN_POINT('',(2.305,-3.74122974434878,0.5));
#34101=CARTESIAN_POINT('',(2.2925,-3.74122974434878,0.5125));
#34102=CARTESIAN_POINT('Origin',(2.16,-3.74122974434878,0.5));
#34103=CARTESIAN_POINT('Origin',(1.95,-3.74122974434878,0.5));
#34104=CARTESIAN_POINT('Origin',(-2.16,-3.74122974434877,1.4125));
#34105=CARTESIAN_POINT('',(-2.04,-3.74122974434877,1.375));
#34106=CARTESIAN_POINT('',(-2.0275,-3.74122974434877,1.4125));
#34107=CARTESIAN_POINT('Origin',(-2.16,-3.74122974434877,1.375));
#34108=CARTESIAN_POINT('Origin',(-2.16,-3.74122974434877,0.95));
#34109=CARTESIAN_POINT('',(-2.04,-3.74122974434877,0.525));
#34110=CARTESIAN_POINT('',(-2.04,-3.74122974434877,0.95));
#34111=CARTESIAN_POINT('Origin',(-2.16,-3.74122974434877,0.525));
#34112=CARTESIAN_POINT('Origin',(-2.16,-3.74122974434877,0.5125));
#34113=CARTESIAN_POINT('',(-2.015,-3.74122974434877,0.5));
#34114=CARTESIAN_POINT('',(-2.0275,-3.74122974434877,0.5125));
#34115=CARTESIAN_POINT('Origin',(-2.16,-3.74122974434877,0.5));
#34116=CARTESIAN_POINT('Origin',(-2.37,-3.74122974434877,0.5));
#34117=CARTESIAN_POINT('Origin',(-4.32,5.29047417231657E-16,1.4125));
#34118=CARTESIAN_POINT('',(-4.2,5.14351655641888E-16,1.375));
#34119=CARTESIAN_POINT('',(-4.1875,5.12820847142954E-16,1.4125));
#34120=CARTESIAN_POINT('Origin',(-4.32,5.29047417231657E-16,1.375));
#34121=CARTESIAN_POINT('Origin',(-4.32,5.29047417231657E-16,0.95));
#34122=CARTESIAN_POINT('',(-4.2,5.14351655641888E-16,0.525));
#34123=CARTESIAN_POINT('',(-4.2,5.14351655641888E-16,0.95));
#34124=CARTESIAN_POINT('Origin',(-4.32,5.29047417231657E-16,0.525));
#34125=CARTESIAN_POINT('Origin',(-4.32,5.29047417231657E-16,0.5125));
#34126=CARTESIAN_POINT('',(-4.175,5.1129003864402E-16,0.5));
#34127=CARTESIAN_POINT('',(-4.1875,5.12820847142954E-16,0.5125));
#34128=CARTESIAN_POINT('Origin',(-4.32,5.29047417231657E-16,0.5));
#34129=CARTESIAN_POINT('Origin',(-4.53,5.29047417231657E-16,0.5));
#34130=CARTESIAN_POINT('Origin',(-2.16,3.74122974434878,1.4125));
#34131=CARTESIAN_POINT('',(-2.04,3.74122974434878,1.375));
#34132=CARTESIAN_POINT('',(-2.0275,3.74122974434878,1.4125));
#34133=CARTESIAN_POINT('Origin',(-2.16,3.74122974434878,1.375));
#34134=CARTESIAN_POINT('Origin',(-2.16,3.74122974434878,0.95));
#34135=CARTESIAN_POINT('',(-2.04,3.74122974434878,0.525));
#34136=CARTESIAN_POINT('',(-2.04,3.74122974434878,0.95));
#34137=CARTESIAN_POINT('Origin',(-2.16,3.74122974434878,0.525));
#34138=CARTESIAN_POINT('Origin',(-2.16,3.74122974434878,0.5125));
#34139=CARTESIAN_POINT('',(-2.015,3.74122974434878,0.5));
#34140=CARTESIAN_POINT('',(-2.0275,3.74122974434878,0.5125));
#34141=CARTESIAN_POINT('Origin',(-2.16,3.74122974434878,0.5));
#34142=CARTESIAN_POINT('Origin',(-2.37,3.74122974434878,0.5));
#34143=CARTESIAN_POINT('Origin',(2.16,3.74122974434878,1.4125));
#34144=CARTESIAN_POINT('',(2.28,3.74122974434878,1.375));
#34145=CARTESIAN_POINT('',(2.2925,3.74122974434878,1.4125));
#34146=CARTESIAN_POINT('Origin',(2.16,3.74122974434878,1.375));
#34147=CARTESIAN_POINT('Origin',(2.16,3.74122974434878,0.95));
#34148=CARTESIAN_POINT('',(2.28,3.74122974434878,0.525));
#34149=CARTESIAN_POINT('',(2.28,3.74122974434878,0.95));
#34150=CARTESIAN_POINT('Origin',(2.16,3.74122974434878,0.525));
#34151=CARTESIAN_POINT('Origin',(2.16,3.74122974434878,0.5125));
#34152=CARTESIAN_POINT('',(2.305,3.74122974434878,0.5));
#34153=CARTESIAN_POINT('',(2.2925,3.74122974434878,0.5125));
#34154=CARTESIAN_POINT('Origin',(2.16,3.74122974434878,0.5));
#34155=CARTESIAN_POINT('Origin',(1.95,3.74122974434878,0.5));
#34156=CARTESIAN_POINT('Origin',(4.32,0.,1.4125));
#34157=CARTESIAN_POINT('',(4.44,-1.46957615897682E-17,1.375));
#34158=CARTESIAN_POINT('',(4.4525,-1.62265700887025E-17,1.4125));
#34159=CARTESIAN_POINT('Origin',(4.32,0.,1.375));
#34160=CARTESIAN_POINT('Origin',(4.32,0.,0.95));
#34161=CARTESIAN_POINT('',(4.44,-1.46957615897683E-17,0.525));
#34162=CARTESIAN_POINT('',(4.44,-1.46957615897683E-17,0.95));
#34163=CARTESIAN_POINT('Origin',(4.32,0.,0.525));
#34164=CARTESIAN_POINT('Origin',(4.32,0.,0.5125));
#34165=CARTESIAN_POINT('',(4.465,-1.77573785876367E-17,0.5));
#34166=CARTESIAN_POINT('',(4.4525,-1.62265700887025E-17,0.5125));
#34167=CARTESIAN_POINT('Origin',(4.32,0.,0.5));
#34168=CARTESIAN_POINT('Origin',(4.11,0.,0.5));
#34169=CARTESIAN_POINT('Origin',(0.,0.,1.98));
#34170=CARTESIAN_POINT('',(4.095,5.01492864250841E-16,1.96));
#34171=CARTESIAN_POINT('',(4.075,4.99043570652547E-16,1.98));
#34172=CARTESIAN_POINT('',(-4.095,-5.01492864250841E-16,1.96));
#34173=CARTESIAN_POINT('Origin',(0.,0.,1.96));
#34174=CARTESIAN_POINT('Origin',(0.,0.,1.96));
#34175=CARTESIAN_POINT('Origin',(0.,0.,1.7));
#34176=CARTESIAN_POINT('',(-4.095,-5.01492864250841E-16,1.7));
#54960=UNCERTAINTY_MEASURE_WITH_UNIT(LENGTH_MEASURE(0.001),#55003,
'DISTANCE_ACCURACY_VALUE',
'Maximum model space distance between geometric entities at asserted c
onnectivities');
#54980=UNCERTAINTY_MEASURE_WITH_UNIT(LENGTH_MEASURE(0.001),#55003,
'DISTANCE_ACCURACY_VALUE',
'Maximum model space distance between geometric entities at asserted c
onnectivities');
#54982=(
GEOMETRIC_REPRESENTATION_CONTEXT(3)
GLOBAL_UNCERTAINTY_ASSIGNED_CONTEXT((#54960))
GLOBAL_UNIT_ASSIGNED_CONTEXT((#55003,#55005,#55006))
REPRESENTATION_CONTEXT('','3D')
);
#55002=(
GEOMETRIC_REPRESENTATION_CONTEXT(3)
GLOBAL_UNCERTAINTY_ASSIGNED_CONTEXT((#54980))
GLOBAL_UNIT_ASSIGNED_CONTEXT((#55003,#55005,#55006))
REPRESENTATION_CONTEXT('','3D')
);
#55003=(
LENGTH_UNIT()
NAMED_UNIT(*)
SI_UNIT(.CENTI.,.METRE.)
);
#55005=(
NAMED_UNIT(*)
PLANE_ANGLE_UNIT()
SI_UNIT($,.RADIAN.)
);
#55006=(
NAMED_UNIT(*)
SI_UNIT($,.STERADIAN.)
SOLID_ANGLE_UNIT()
);
#55008=SHAPE_DEFINITION_REPRESENTATION(#55029,#55104);
#55029=PRODUCT_DEFINITION_SHAPE('',$,#55126);
#55104=SHAPE_REPRESENTATION('',(#24771),#54982);
#55124=PRODUCT_DEFINITION_CONTEXT('part definition',#55189,'design');
#55126=PRODUCT_DEFINITION('2026-10-18-23-35-47-869',
'01_Rear_End_Cap_D95',#55147,#55124);
#55147=PRODUCT_DEFINITION_FORMATION('',$,#55192);
#55189=APPLICATION_CONTEXT(
'Core Data for Automotive Mechanical Design Process');
#55190=PRODUCT_CONTEXT('part definition',#55189,'mechanical');
#55192=PRODUCT('2026-10-18-23-35-47-869','01_Rear_End_Cap_D95',$,(#55190));
#55366=COLOUR_RGB('Light Blue',0.38,0.62,0.78);
#55367=FILL_AREA_STYLE_COLOUR('',#55366);
#55368=FILL_AREA_STYLE('',(#55367));
#55369=SURFACE_STYLE_FILL_AREA(#55368);
#55370=SURFACE_SIDE_STYLE('',(#55369));
#55371=SURFACE_STYLE_USAGE(.BOTH.,#55370);
#55372=PRESENTATION_STYLE_ASSIGNMENT((#55371));
ENDSEC;
END-ISO-10303-21;
